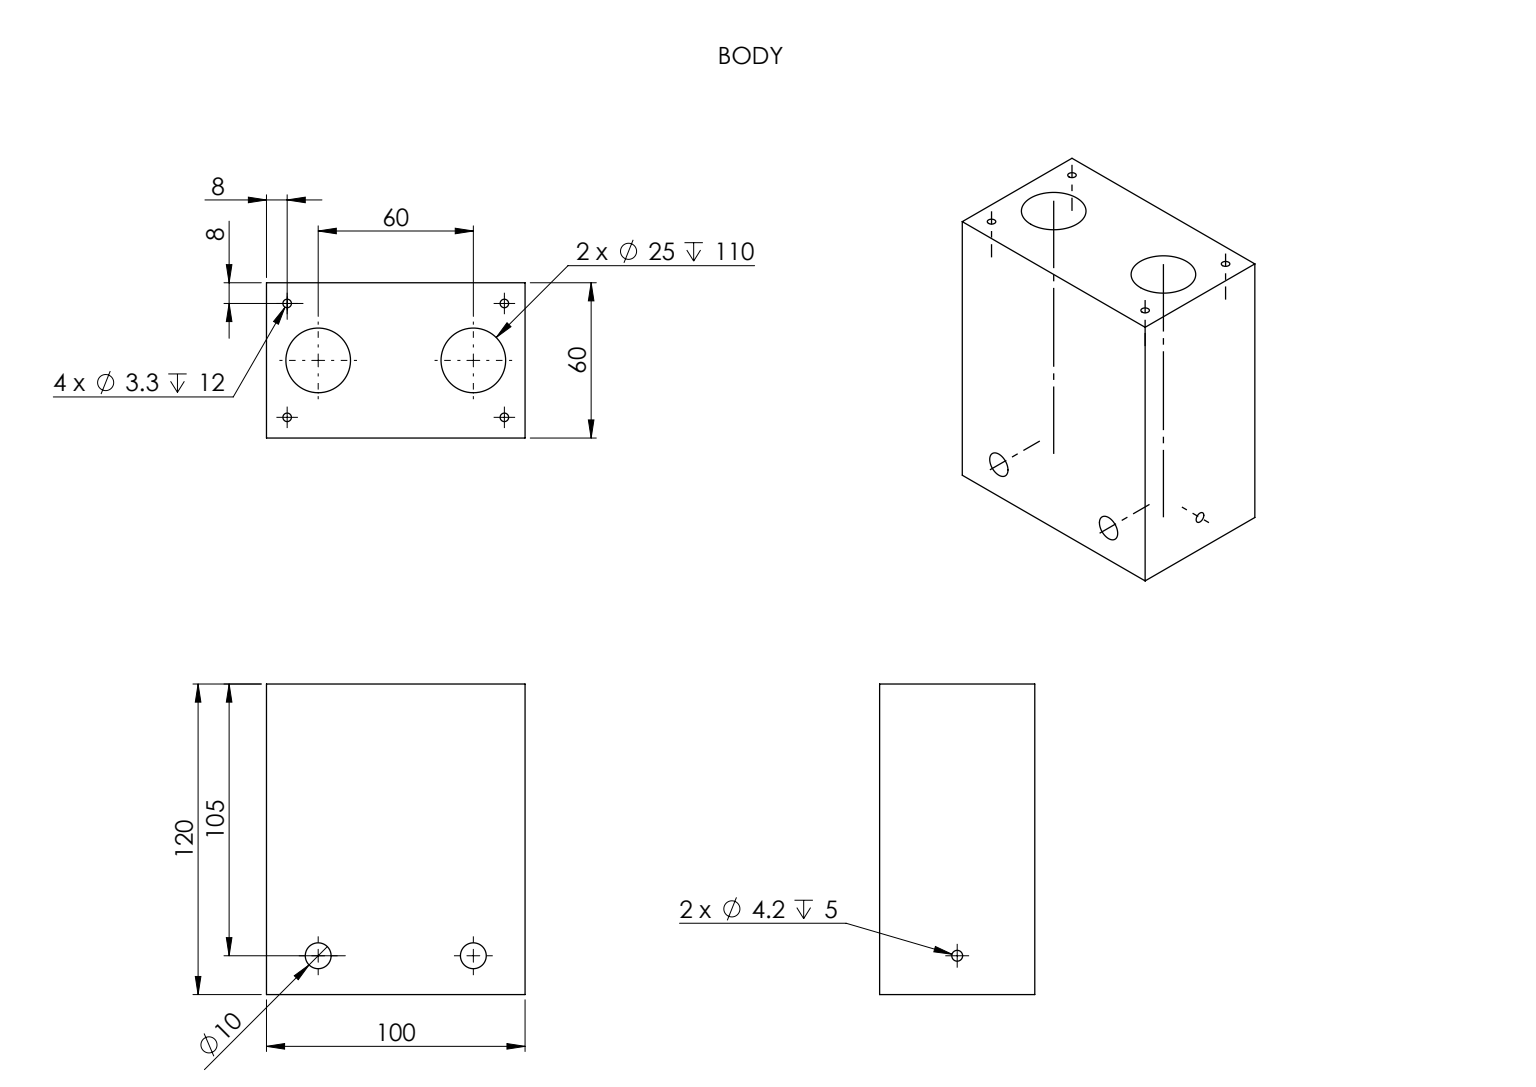
ISO-10303-21;
HEADER;
FILE_DESCRIPTION (('STEP AP214'),
    '1' );
FILE_NAME ('Body.step',
    '2026-09-29T11:11:29',
    ( '' ),
    ( '' ),
    'SwSTEP 2.0',
    'SolidWorks 2026',
    '' );
FILE_SCHEMA (( 'AUTOMOTIVE_DESIGN' ));
ENDSEC;

DATA;
#5=CARTESIAN_POINT ( 'NONE',  ( 42.00000000000000711, 48.00000000000002842, -23.64999999999992042 ) ) ;
#32=CIRCLE ( 'NONE', #4965, 12.49999999999997335 ) ;
#39=STYLED_ITEM ( 'NONE', ( #683 ), #2810 ) ;
#44=CARTESIAN_POINT ( 'NONE',  ( 25.66305258423476943, -47.50955795526802206, 11.72510588894413530 ) ) ;
#45=CARTESIAN_POINT ( 'NONE',  ( -41.99999999999996447, 48.00000000000002842, 22.00000000000000000 ) ) ;
#46=CONICAL_SURFACE ( 'NONE', #7936, 12.49999999999996980, 1.029744258676651869 ) ;
#53=CARTESIAN_POINT ( 'NONE',  ( 26.69566991153659785, -41.23356742411069575, 12.05770814628967535 ) ) ;
#54=DIRECTION ( 'NONE',  ( 1.000000000000000000, 0.000000000000000000, 0.000000000000000000 ) ) ;
#58=VERTEX_POINT ( 'NONE', #8160 ) ;
#70=CARTESIAN_POINT ( 'NONE',  ( -30.00000000000000000, 60.00000000000002842, 0.000000000000000000 ) ) ;
#76=ADVANCED_FACE ( 'NONE', ( #1450 ), #4832, .F. ) ;
#87=ADVANCED_FACE ( 'NONE', ( #4979 ), #2915, .F. ) ;
#90=UNCERTAINTY_MEASURE_WITH_UNIT (LENGTH_MEASURE( 1.000000000000000082E-05 ), #727, 'distance_accuracy_value', 'NONE');
#92=DIRECTION ( 'NONE',  ( -0.000000000000000000, 1.000000000000000000, -0.000000000000000000 ) ) ;
#99=EDGE_CURVE ( 'NONE', #4623, #6070, #4272, .T. ) ;
#100=CARTESIAN_POINT ( 'NONE',  ( -30.00000000000000000, -40.00000000000002132, 12.49999999999998046 ) ) ;
#101=CIRCLE ( 'NONE', #1224, 4.999999999999973355 ) ;
#104=CARTESIAN_POINT ( 'NONE',  ( -49.99999999999997158, -59.99999999999997158, -30.00000000000000000 ) ) ;
#113=ORIENTED_EDGE ( 'NONE', *, *, #1064, .F. ) ;
#125=DIRECTION ( 'NONE',  ( -0.000000000000000000, 1.000000000000000000, -0.000000000000000000 ) ) ;
#139=EDGE_LOOP ( 'NONE', ( #1708, #6887, #7126, #967 ) ) ;
#140=CARTESIAN_POINT ( 'NONE',  ( 0.000000000000000000, 0.000000000000000000, -30.00000000000000000 ) ) ;
#144=CARTESIAN_POINT ( 'NONE',  ( -25.51828610110682405, -42.77717578641267693, 11.66923617342549413 ) ) ;
#145=CARTESIAN_POINT ( 'NONE',  ( 45.00000000000003553, -44.99999999999997158, 0.000000000000000000 ) ) ;
#150=EDGE_LOOP ( 'NONE', ( #1097, #2734, #1435, #2240, #218 ) ) ;
#151=LINE ( 'NONE', #8229, #3888 ) ;
#158=EDGE_CURVE ( 'NONE', #8668, #1053, #2208, .T. ) ;
#161=DIRECTION ( 'NONE',  ( 0.000000000000000000, 0.000000000000000000, 1.000000000000000000 ) ) ;
#187=CARTESIAN_POINT ( 'NONE',  ( 29.34107419296792685, -40.03249052150653142, 12.48689449661282858 ) ) ;
#205=CARTESIAN_POINT ( 'NONE',  ( -25.16271839757670747, -46.30802241892378390, 11.52630626327735364 ) ) ;
#207=VERTEX_POINT ( 'NONE', #7881 ) ;
#210=ORIENTED_EDGE ( 'NONE', *, *, #267, .T. ) ;
#218=ORIENTED_EDGE ( 'NONE', *, *, #2863, .T. ) ;
#228=CARTESIAN_POINT ( 'NONE',  ( 25.51351754887333101, -42.76835092305877595, 11.66791272636411847 ) ) ;
#235=CARTESIAN_POINT ( 'NONE',  ( 50.00000000000002842, -44.99999999999997158, 0.000000000000000000 ) ) ;
#236=ORIENTED_EDGE ( 'NONE', *, *, #746, .T. ) ;
#247=CARTESIAN_POINT ( 'NONE',  ( -49.99999999999997158, 60.00000000000002842, 30.00000000000000000 ) ) ;
#249=ORIENTED_EDGE ( 'NONE', *, *, #158, .T. ) ;
#253=ORIENTED_EDGE ( 'NONE', *, *, #4306, .F. ) ;
#260=ORIENTED_EDGE ( 'NONE', *, *, #8374, .T. ) ;
#267=EDGE_CURVE ( 'NONE', #4999, #1695, #7837, .T. ) ;
#268=DIRECTION ( 'NONE',  ( -0.000000000000000000, 1.000000000000000000, -0.000000000000000000 ) ) ;
#279=ORIENTED_EDGE ( 'NONE', *, *, #4946, .T. ) ;
#290=FACE_OUTER_BOUND ( 'NONE', #2679, .T. ) ;
#302=STYLED_ITEM ( 'NONE', ( #2499 ), #2657 ) ;
#313=CARTESIAN_POINT ( 'NONE',  ( 50.00000000000002842, -44.99999999999997158, 0.000000000000000000 ) ) ;
#327=CARTESIAN_POINT ( 'NONE',  ( 42.00000000000000711, 60.00000000000002842, -20.34999999999992326 ) ) ;
#328=CARTESIAN_POINT ( 'NONE',  ( 25.00000000000004263, -44.99999999999995737, 11.45643923738958314 ) ) ;
#337=ORIENTED_EDGE ( 'NONE', *, *, #267, .F. ) ;
#346=ORIENTED_EDGE ( 'NONE', *, *, #5233, .F. ) ;
#349=CARTESIAN_POINT ( 'NONE',  ( 42.00000000000000711, 60.00000000000002842, -21.99999999999992184 ) ) ;
#356=DIRECTION ( 'NONE',  ( 0.000000000000000000, 0.000000000000000000, 1.000000000000000000 ) ) ;
#358=DIRECTION ( 'NONE',  ( -0.000000000000000000, 1.000000000000000000, -0.000000000000000000 ) ) ;
#366=DIRECTION ( 'NONE',  ( 0.000000000000000000, 0.000000000000000000, 1.000000000000000000 ) ) ;
#372=( LENGTH_UNIT ( ) NAMED_UNIT ( * ) SI_UNIT ( .MILLI., .METRE. ) );
#373=ORIENTED_EDGE ( 'NONE', *, *, #4139, .T. ) ;
#383=CONICAL_SURFACE ( 'NONE', #2372, 1.649999999999998579, 1.029744258676653645 ) ;
#395=EDGE_CURVE ( 'NONE', #6859, #7279, #4993, .T. ) ;
#403=CARTESIAN_POINT ( 'NONE',  ( 33.05708889405230622, -41.03022111473440958, 12.12354317000652770 ) ) ;
#414=ORIENTED_EDGE ( 'NONE', *, *, #7534, .T. ) ;
#417=CARTESIAN_POINT ( 'NONE',  ( -30.33426447602078113, -49.99999999999997868, 12.49999999999998046 ) ) ;
#424=ORIENTED_EDGE ( 'NONE', *, *, #7210, .T. ) ;
#429=CYLINDRICAL_SURFACE ( 'NONE', #2354, 1.649999999999998579 ) ;
#433=DIRECTION ( 'NONE',  ( -0.000000000000000000, 1.000000000000000000, -0.000000000000000000 ) ) ;
#443=CARTESIAN_POINT ( 'NONE',  ( 33.76876201869192329, -41.69806059905381090, 11.92074493419279158 ) ) ;
#447=CARTESIAN_POINT ( 'NONE',  ( -50.00000000000002842, -44.99999999999997158, 0.000000000000000000 ) ) ;
#448=COLOUR_RGB ( '', 0.66274510, 0.83137255, 0.94901961) ;
#451=LINE ( 'NONE', #2589, #1885 ) ;
#454=AXIS2_PLACEMENT_3D ( 'NONE', #6879, #842, #8222 ) ;
#458=CARTESIAN_POINT ( 'NONE',  ( -30.66228279038040228, -49.96682304584954437, 12.48662461771948529 ) ) ;
#461=DIRECTION ( 'NONE',  ( -0.000000000000000000, 1.000000000000000000, -0.000000000000000000 ) ) ;
#467=ORIENTED_EDGE ( 'NONE', *, *, #5580, .T. ) ;
#481=VECTOR ( 'NONE', #6597, 1000.000000000000000 ) ;
#491=ORIENTED_EDGE ( 'NONE', *, *, #6060, .T. ) ;
#495=EDGE_CURVE ( 'NONE', #3168, #8538, #1819, .T. ) ;
#498=ORIENTED_EDGE ( 'NONE', *, *, #6490, .F. ) ;
#500=CARTESIAN_POINT ( 'NONE',  ( -34.82961390090871134, -46.30459253935130448, 11.52942094433410425 ) ) ;
#518=CARTESIAN_POINT ( 'NONE',  ( -41.99999999999996447, 48.00000000000002842, 20.35000000000000142 ) ) ;
#523=ORIENTED_EDGE ( 'NONE', *, *, #1974, .F. ) ;
#529=CARTESIAN_POINT ( 'NONE',  ( 30.00000000000000000, -49.99999999999997158, -1.102182119232617753E-14 ) ) ;
#533=ADVANCED_FACE ( 'NONE', ( #4459 ), #1022, .F. ) ;
#534=CARTESIAN_POINT ( 'NONE',  ( 30.00000000000000000, 60.00000000000002842, -1.102182119232617753E-14 ) ) ;
#548=CARTESIAN_POINT ( 'NONE',  ( 33.76617411639087152, -48.30471456237972205, 11.92153802757354342 ) ) ;
#550=EDGE_LOOP ( 'NONE', ( #7307, #8387, #6188 ) ) ;
#556=B_SPLINE_CURVE_WITH_KNOTS ( 'NONE', 3,
 ( #4547, #3887, #5995, #8125, #5416, #2084, #2749, #4769, #1411, #7454, #4108, #44, #6786, #749, #6087, #3810, #3729, #1657, #2452, #328 ),
 .UNSPECIFIED., .F., .F.,
 ( 4, 2, 2, 2, 2, 2, 2, 2, 2, 4 ),
 ( 2.088883680402604765E-17, 0.0009878455431464048045, 0.001975691086292788792, 0.002963536629439172780, 0.003951382172585556768, 0.004939227715731940756, 0.005927073258878324744, 0.006420996030451506763, 0.006914918802024689649, 0.007902764345171071902 ),
 .UNSPECIFIED. ) ;
#567=EDGE_LOOP ( 'NONE', ( #498, #2058, #5139, #6935, #113, #2462 ) ) ;
#579=AXIS2_PLACEMENT_3D ( 'NONE', #3617, #8335, #2961 ) ;
#589=MECHANICAL_DESIGN_GEOMETRIC_PRESENTATION_REPRESENTATION('',(#39),#3149);
#597=VECTOR ( 'NONE', #1210, 1000.000000000000000 ) ;
#605=VECTOR ( 'NONE', #8413, 1000.000000000000000 ) ;
#620=DIRECTION ( 'NONE',  ( -0.000000000000000000, 1.000000000000000000, -0.000000000000000000 ) ) ;
#625=EDGE_LOOP ( 'NONE', ( #5700, #4753, #2629, #4443 ) ) ;
#626=CARTESIAN_POINT ( 'NONE',  ( -50.00000000000002842, -44.99999999999997158, 2.099999999999997868 ) ) ;
#637=FILL_AREA_STYLE_COLOUR ( '', #448 ) ;
#638=LINE ( 'NONE', #4044, #1797 ) ;
#645=CIRCLE ( 'NONE', #5579, 1.649999999999998579 ) ;
#654=AXIS2_PLACEMENT_3D ( 'NONE', #7280, #754, #5374 ) ;
#668=DIRECTION ( 'NONE',  ( 0.000000000000000000, 0.000000000000000000, -1.000000000000000000 ) ) ;
#671=DIRECTION ( 'NONE',  ( -0.000000000000000000, 1.000000000000000000, -0.000000000000000000 ) ) ;
#674=LINE ( 'NONE', #8046, #3482 ) ;
#679=CLOSED_SHELL ( 'NONE', ( #7354, #6229, #8350, #1433, #4093, #6520, #7720, #1560, #7628, #4521, #4016, #3800, #5743, #3822, #7621, #4055, #7669, #4185, #6558, #1536, #3196, #3679, #1549, #5972, #76, #87, #7313, #7419, #7801, #4973, #8008, #2481, #4022, #3615, #4856, #2349, #5957, #8496, #3760, #533, #2845, #7262 ) ) ;
#683=PRESENTATION_STYLE_ASSIGNMENT (( #2596 ) ) ;
#686=CARTESIAN_POINT ( 'NONE',  ( 32.51701891408353617, -49.33233869400790184, 12.24706002614420264 ) ) ;
#699=CONICAL_SURFACE ( 'NONE', #7040, 12.49999999999997335, 1.029744258676651869 ) ;
#708=DIRECTION ( 'NONE',  ( 1.049727191138618079E-16, 0.5150380749100549327, -0.8571673007021118895 ) ) ;
#711=CARTESIAN_POINT ( 'NONE',  ( -41.99999999999996447, 47.00857997860455129, -22.00000000000000000 ) ) ;
#712=DIRECTION ( 'NONE',  ( 0.000000000000000000, 0.000000000000000000, 1.000000000000000000 ) ) ;
#724=VERTEX_POINT ( 'NONE', #2388 ) ;
#727=( LENGTH_UNIT ( ) NAMED_UNIT ( * ) SI_UNIT ( .MILLI., .METRE. ) );
#728=DIRECTION ( 'NONE',  ( 1.049727191138617093E-16, 0.5150380749100563760, -0.8571673007021110013 ) ) ;
#735=EDGE_CURVE ( 'NONE', #1784, #5916, #4447, .T. ) ;
#739=DIRECTION ( 'NONE',  ( 0.000000000000000000, 0.000000000000000000, 1.000000000000000000 ) ) ;
#746=EDGE_CURVE ( 'NONE', #2486, #6385, #6425, .T. ) ;
#749=CARTESIAN_POINT ( 'NONE',  ( 25.32221232802729460, -46.77334385938312522, 11.59192968702632065 ) ) ;
#754=DIRECTION ( 'NONE',  ( -0.000000000000000000, -0.000000000000000000, 1.000000000000000000 ) ) ;
#759=FACE_OUTER_BOUND ( 'NONE', #5969, .T. ) ;
#762=CYLINDRICAL_SURFACE ( 'NONE', #8087, 1.649999999999998579 ) ;
#766=EDGE_LOOP ( 'NONE', ( #3607, #2663 ) ) ;
#778=EDGE_CURVE ( 'NONE', #6845, #1128, #7172, .T. ) ;
#784=DIRECTION ( 'NONE',  ( 0.000000000000000000, 0.000000000000000000, 1.000000000000000000 ) ) ;
#801=VECTOR ( 'NONE', #7421, 1000.000000000000000 ) ;
#803=EDGE_CURVE ( 'NONE', #4035, #3309, #1727, .T. ) ;
#805=CARTESIAN_POINT ( 'NONE',  ( 29.67102067851989844, -40.00000000000000000, 12.49999999999996980 ) ) ;
#820=LINE ( 'NONE', #2774, #3625 ) ;
#823=FACE_BOUND ( 'NONE', #7168, .T. ) ;
#829=DIRECTION ( 'NONE',  ( 0.000000000000000000, 0.000000000000000000, 1.000000000000000000 ) ) ;
#842=DIRECTION ( 'NONE',  ( 0.000000000000000000, 0.000000000000000000, 1.000000000000000000 ) ) ;
#845=CARTESIAN_POINT ( 'NONE',  ( 25.16326641152763344, -43.69081521296084958, 11.52653374317613455 ) ) ;
#846=DIRECTION ( 'NONE',  ( -0.000000000000000000, 1.000000000000000000, -0.000000000000000000 ) ) ;
#857=AXIS2_PLACEMENT_3D ( 'NONE', #3752, #2969, #5644 ) ;
#868=EDGE_LOOP ( 'NONE', ( #8063, #1620, #467 ) ) ;
#880=VECTOR ( 'NONE', #8032, 1000.000000000000000 ) ;
#883=CARTESIAN_POINT ( 'NONE',  ( -30.00000000000000000, 60.00000000000002842, 12.49999999999998757 ) ) ;
#884=PRODUCT_CONTEXT ( 'NONE', #2293, 'mechanical' ) ;
#885=CARTESIAN_POINT ( 'NONE',  ( -41.99999999999996447, 48.00000000000002842, -23.64999999999999858 ) ) ;
#897=EDGE_LOOP ( 'NONE', ( #6623, #5315 ) ) ;
#906=DIRECTION ( 'NONE',  ( -1.000000000000000000, -0.000000000000000000, -0.000000000000000000 ) ) ;
#907=CARTESIAN_POINT ( 'NONE',  ( -34.33209868862994796, -42.48249851487850748, 11.72687238757476003 ) ) ;
#911=EDGE_CURVE ( 'NONE', #6845, #2769, #1890, .T. ) ;
#912=VERTEX_POINT ( 'NONE', #6680 ) ;
#915=ORIENTED_EDGE ( 'NONE', *, *, #5570, .F. ) ;
#919=LINE ( 'NONE', #1532, #6968 ) ;
#925=CIRCLE ( 'NONE', #7677, 1.649999999999998579 ) ;
#935=CARTESIAN_POINT ( 'NONE',  ( -26.02663761693602495, -41.94765302695305564, 11.85321826485150432 ) ) ;
#947=CIRCLE ( 'NONE', #3762, 1.649999999999998579 ) ;
#962=DIRECTION ( 'NONE',  ( -1.000000000000000000, -0.000000000000000000, -0.000000000000000000 ) ) ;
#967=ORIENTED_EDGE ( 'NONE', *, *, #158, .F. ) ;
#971=CARTESIAN_POINT ( 'NONE',  ( -41.99999999999996447, 60.00000000000002842, 20.35000000000000142 ) ) ;
#983=ORIENTED_EDGE ( 'NONE', *, *, #2920, .F. ) ;
#988=B_SPLINE_CURVE_WITH_KNOTS ( 'NONE', 3,
 ( #3772, #7077, #5751, #3162, #1036, #2329, #5007, #7696, #3075, #403, #8450, #443, #5836, #2492, #5173, #4512, #8089, #7329, #1955, #5292, #8613, #1873 ),
 .UNSPECIFIED., .F., .F.,
 ( 4, 2, 2, 2, 2, 2, 2, 2, 2, 2, 4 ),
 ( 0.01579945264986103853, 0.01629290087626464323, 0.01678634910266824792, 0.01777324555547545731, 0.01876014200828266323, 0.01974703846108986915, 0.02073393491389707508, 0.02122738314030068324, 0.02172083136670428793, 0.02270772781951150079, 0.02369462427231871365 ),
 .UNSPECIFIED. ) ;
#991=DIRECTION ( 'NONE',  ( -0.000000000000000000, 1.000000000000000000, -0.000000000000000000 ) ) ;
#992=CARTESIAN_POINT ( 'NONE',  ( -26.23382588360912848, -48.30471456237976469, 11.92153802757356118 ) ) ;
#995=EDGE_CURVE ( 'NONE', #5982, #8204, #1392, .T. ) ;
#1005=DIRECTION ( 'NONE',  ( -1.000000000000000000, 0.000000000000000000, 0.000000000000000000 ) ) ;
#1008=EDGE_CURVE ( 'NONE', #6235, #8538, #3206, .T. ) ;
#1016=CIRCLE ( 'NONE', #1730, 12.49999999999998401 ) ;
#1018=EDGE_CURVE ( 'NONE', #2059, #1305, #638, .T. ) ;
#1022=CYLINDRICAL_SURFACE ( 'NONE', #3219, 2.099999999999997868 ) ;
#1024=DIRECTION ( 'NONE',  ( 0.000000000000000000, 0.000000000000000000, 1.000000000000000000 ) ) ;
#1026=LINE ( 'NONE', #3103, #1095 ) ;
#1029=ORIENTED_EDGE ( 'NONE', *, *, #2094, .F. ) ;
#1036=CARTESIAN_POINT ( 'NONE',  ( 30.82435085130693153, -40.06565635038678863, 12.47384660903967735 ) ) ;
#1049=CYLINDRICAL_SURFACE ( 'NONE', #6547, 1.649999999999998579 ) ;
#1051=CARTESIAN_POINT ( 'NONE',  ( 50.00000000000002842, -59.99999999999997158, 30.00000000000000000 ) ) ;
#1053=VERTEX_POINT ( 'NONE', #2859 ) ;
#1055=EDGE_CURVE ( 'NONE', #6557, #4874, #820, .T. ) ;
#1062=PRODUCT ( 'Body', 'Body', '', ( #884 ) ) ;
#1064=EDGE_CURVE ( 'NONE', #7279, #8149, #6180, .T. ) ;
#1067=CARTESIAN_POINT ( 'NONE',  ( 42.00000000000000711, 48.00000000000002842, 21.99999999999992184 ) ) ;
#1069=DIRECTION ( 'NONE',  ( 0.000000000000000000, 0.000000000000000000, 1.000000000000000000 ) ) ;
#1076=VECTOR ( 'NONE', #3796, 1000.000000000000000 ) ;
#1081=CARTESIAN_POINT ( 'NONE',  ( -49.99999999999997158, -59.99999999999997158, 30.00000000000000000 ) ) ;
#1089=VECTOR ( 'NONE', #1578, 1000.000000000000000 ) ;
#1091=CARTESIAN_POINT ( 'NONE',  ( -30.00000000000000000, -49.99999999999997158, 12.49999999999997335 ) ) ;
#1095=VECTOR ( 'NONE', #5784, 1000.000000000000000 ) ;
#1097=ORIENTED_EDGE ( 'NONE', *, *, #3505, .F. ) ;
#1100=VERTEX_POINT ( 'NONE', #4132 ) ;
#1121=CARTESIAN_POINT ( 'NONE',  ( -26.02892847301724544, -48.05549307397419767, 11.85400291056945576 ) ) ;
#1124=EDGE_LOOP ( 'NONE', ( #7069, #6657, #3793 ) ) ;
#1128=VERTEX_POINT ( 'NONE', #4173 ) ;
#1134=CARTESIAN_POINT ( 'NONE',  ( 42.00000000000000711, 48.00000000000002842, -20.34999999999992326 ) ) ;
#1142=DIRECTION ( 'NONE',  ( 0.000000000000000000, 0.000000000000000000, 1.000000000000000000 ) ) ;
#1152=EDGE_LOOP ( 'NONE', ( #2553, #2380, #260, #2838 ) ) ;
#1165=CIRCLE ( 'NONE', #5378, 4.999999999999969802 ) ;
#1173=ORIENTED_EDGE ( 'NONE', *, *, #7210, .F. ) ;
#1176=CARTESIAN_POINT ( 'NONE',  ( -34.99999999999997868, -45.33027059730886066, 11.45643923738958847 ) ) ;
#1179=DIRECTION ( 'NONE',  ( 1.049727191138617093E-16, 0.5150380749100563760, -0.8571673007021110013 ) ) ;
#1187=CARTESIAN_POINT ( 'NONE',  ( 30.00000000000001421, -49.99999999999997158, 12.49999999999995914 ) ) ;
#1190=CARTESIAN_POINT ( 'NONE',  ( -34.99999999999997868, -45.00000000000000000, 11.45643923738958847 ) ) ;
#1201=DIRECTION ( 'NONE',  ( -0.5150380749100560429, 1.049727191138617340E-16, -0.8571673007021112234 ) ) ;
#1206=CARTESIAN_POINT ( 'NONE',  ( 30.00000000000000000, 60.00000000000002842, -1.102182119232617753E-14 ) ) ;
#1210=DIRECTION ( 'NONE',  ( 0.000000000000000000, 0.5150380749100549327, 0.8571673007021118895 ) ) ;
#1224=AXIS2_PLACEMENT_3D ( 'NONE', #5201, #3231, #6698 ) ;
#1225=EDGE_LOOP ( 'NONE', ( #7122, #8635, #4534, #6637, #1029, #5348 ) ) ;
#1236=CARTESIAN_POINT ( 'NONE',  ( -49.99999999999997158, -59.99999999999997158, -30.00000000000000000 ) ) ;
#1238=ORIENTED_EDGE ( 'NONE', *, *, #4139, .F. ) ;
#1242=CARTESIAN_POINT ( 'NONE',  ( -50.00000000000002842, -44.99999999999997158, 0.000000000000000000 ) ) ;
#1246=CARTESIAN_POINT ( 'NONE',  ( 42.00000000000000711, 60.00000000000002842, 21.99999999999992184 ) ) ;
#1253=ORIENTED_EDGE ( 'NONE', *, *, #4029, .F. ) ;
#1257=DIRECTION ( 'NONE',  ( -0.000000000000000000, 1.000000000000000000, -0.000000000000000000 ) ) ;
#1260=ORIENTED_EDGE ( 'NONE', *, *, #4573, .F. ) ;
#1278=ORIENTED_EDGE ( 'NONE', *, *, #3659, .T. ) ;
#1290=ORIENTED_EDGE ( 'NONE', *, *, #3181, .F. ) ;
#1303=CARTESIAN_POINT ( 'NONE',  ( 33.97107152698276877, -48.05549307397414793, 11.85400291056944333 ) ) ;
#1305=VERTEX_POINT ( 'NONE', #5506 ) ;
#1317=AXIS2_PLACEMENT_3D ( 'NONE', #1754, #3775, #7828 ) ;
#1324=CARTESIAN_POINT ( 'NONE',  ( 30.00000000000000000, 60.00000000000002842, -12.49999999999999467 ) ) ;
#1344=SURFACE_SIDE_STYLE ('',( #6065 ) ) ;
#1347=CARTESIAN_POINT ( 'NONE',  ( -30.00000000000000000, -49.99999999999997158, 12.49999999999997335 ) ) ;
#1354=VERTEX_POINT ( 'NONE', #971 ) ;
#1365=B_SPLINE_CURVE_WITH_KNOTS ( 'NONE', 3,
 ( #100, #6269, #6969, #8177, #4869, #4159, #5558, #4243, #4776, #6926, #3506, #5604, #935, #6183, #2889, #144, #5516, #5425, #8225, #8134, #2093, #4377 ),
 .UNSPECIFIED., .F., .F.,
 ( 4, 2, 2, 2, 2, 2, 2, 2, 2, 2, 4 ),
 ( 0.01579945264986107323, 0.01629290087626467792, 0.01678634910266828609, 0.01777324555547549201, 0.01876014200828270140, 0.01974703846108990732, 0.02073393491389711671, 0.02122738314030071100, 0.02172083136670430875, 0.02270772781951152161, 0.02369462427231873447 ),
 .UNSPECIFIED. ) ;
#1372=CYLINDRICAL_SURFACE ( 'NONE', #654, 4.999999999999973355 ) ;
#1379=CARTESIAN_POINT ( 'NONE',  ( 42.00000000000000711, 48.00000000000002842, 21.99999999999992184 ) ) ;
#1382=ORIENTED_EDGE ( 'NONE', *, *, #5368, .F. ) ;
#1392=LINE ( 'NONE', #8630, #8276 ) ;
#1400=ORIENTED_EDGE ( 'NONE', *, *, #3769, .F. ) ;
#1401=EDGE_LOOP ( 'NONE', ( #1260, #6461 ) ) ;
#1411=CARTESIAN_POINT ( 'NONE',  ( 26.68912794345745709, -48.76061935842967898, 12.05589577412331082 ) ) ;
#1412=CARTESIAN_POINT ( 'NONE',  ( 42.00000000000000711, 60.00000000000002842, 20.34999999999992326 ) ) ;
#1420=CARTESIAN_POINT ( 'NONE',  ( 25.00000000000004619, -44.66998333124461595, 11.45643923738958314 ) ) ;
#1422=FACE_OUTER_BOUND ( 'NONE', #4365, .T. ) ;
#1433=ADVANCED_FACE ( 'NONE', ( #2687 ), #7405, .F. ) ;
#1435=ORIENTED_EDGE ( 'NONE', *, *, #5478, .T. ) ;
#1450=FACE_OUTER_BOUND ( 'NONE', #5373, .T. ) ;
#1465=CARTESIAN_POINT ( 'NONE',  ( 27.49109988343930766, -40.67193172067894835, 12.24650812517141674 ) ) ;
#1479=CARTESIAN_POINT ( 'NONE',  ( -32.22066341043710480, -40.51720970344483419, 12.30204028087673862 ) ) ;
#1483=EDGE_LOOP ( 'NONE', ( #1839, #1601, #3000 ) ) ;
#1499=CARTESIAN_POINT ( 'NONE',  ( -41.99999999999996447, 60.00000000000002842, 20.35000000000000142 ) ) ;
#1501=ORIENTED_EDGE ( 'NONE', *, *, #5685, .F. ) ;
#1507=CARTESIAN_POINT ( 'NONE',  ( 26.02887806073490751, -41.94466314146772845, 11.85397847079113731 ) ) ;
#1509=FACE_OUTER_BOUND ( 'NONE', #7442, .T. ) ;
#1525=PLANE ( 'NONE',  #3187 ) ;
#1526=ORIENTED_EDGE ( 'NONE', *, *, #6608, .F. ) ;
#1529=ORIENTED_EDGE ( 'NONE', *, *, #3755, .F. ) ;
#1531=CARTESIAN_POINT ( 'NONE',  ( 42.00000000000000711, 60.00000000000002842, 23.64999999999992042 ) ) ;
#1532=CARTESIAN_POINT ( 'NONE',  ( -50.00000000000002842, -44.99999999999997158, -2.099999999999997868 ) ) ;
#1536=ADVANCED_FACE ( 'NONE', ( #4843, #4796, #4135, #4219, #5577, #4091, #6201 ), #4925, .F. ) ;
#1539=EDGE_CURVE ( 'NONE', #8159, #6416, #3611, .T. ) ;
#1546=EDGE_CURVE ( 'NONE', #4874, #8668, #2062, .T. ) ;
#1548=CIRCLE ( 'NONE', #2830, 1.649999999999998579 ) ;
#1549=ADVANCED_FACE ( 'NONE', ( #823, #2909, #4176 ), #1525, .F. ) ;
#1555=DIRECTION ( 'NONE',  ( 0.000000000000000000, 0.000000000000000000, 1.000000000000000000 ) ) ;
#1560=ADVANCED_FACE ( 'NONE', ( #1568 ), #2357, .F. ) ;
#1565=CARTESIAN_POINT ( 'NONE',  ( -32.07348704419703012, -40.44729329317338795, 12.32776405682971621 ) ) ;
#1568=FACE_OUTER_BOUND ( 'NONE', #1483, .T. ) ;
#1578=DIRECTION ( 'NONE',  ( 1.000000000000000000, 0.000000000000000000, 0.000000000000000000 ) ) ;
#1598=VECTOR ( 'NONE', #3859, 1000.000000000000000 ) ;
#1601=ORIENTED_EDGE ( 'NONE', *, *, #5761, .T. ) ;
#1602=CARTESIAN_POINT ( 'NONE',  ( 50.00000000000002842, -59.99999999999997158, 30.00000000000000000 ) ) ;
#1614=CARTESIAN_POINT ( 'NONE',  ( -26.94596629111760322, -48.97208017019580950, 12.12430375744701827 ) ) ;
#1617=VERTEX_POINT ( 'NONE', #5442 ) ;
#1620=ORIENTED_EDGE ( 'NONE', *, *, #6650, .T. ) ;
#1622=DIRECTION ( 'NONE',  ( -0.000000000000000000, 1.000000000000000000, -0.000000000000000000 ) ) ;
#1623=FACE_OUTER_BOUND ( 'NONE', #5831, .T. ) ;
#1625=CARTESIAN_POINT ( 'NONE',  ( -30.00000000000000000, 60.00000000000002842, -12.49999999999998934 ) ) ;
#1636=CARTESIAN_POINT ( 'NONE',  ( 30.00000000000000000, -49.99999999999997158, -12.49999999999998046 ) ) ;
#1638=AXIS2_PLACEMENT_3D ( 'NONE', #235, #8314, #8308 ) ;
#1643=DIRECTION ( 'NONE',  ( -0.000000000000000000, 1.000000000000000000, -0.000000000000000000 ) ) ;
#1645=DIRECTION ( 'NONE',  ( 1.000000000000000000, 0.000000000000000000, 0.000000000000000000 ) ) ;
#1648=ORIENTED_EDGE ( 'NONE', *, *, #803, .T. ) ;
#1657=CARTESIAN_POINT ( 'NONE',  ( 25.03240331249625328, -45.65721116879221597, 11.47074269425085191 ) ) ;
#1667=ORIENTED_EDGE ( 'NONE', *, *, #1064, .T. ) ;
#1669=CARTESIAN_POINT ( 'NONE',  ( -32.51667136668694269, -49.33273298888241243, 12.24717930254582043 ) ) ;
#1672=CARTESIAN_POINT ( 'NONE',  ( 42.00000000000000711, 60.00000000000002842, -21.99999999999992184 ) ) ;
#1673=CARTESIAN_POINT ( 'NONE',  ( 30.00000000000000000, 60.00000000000002842, -12.49999999999998757 ) ) ;
#1677=EDGE_LOOP ( 'NONE', ( #5190, #1290, #7369, #3341, #3312, #2576 ) ) ;
#1680=DIRECTION ( 'NONE',  ( -1.000000000000000000, -0.000000000000000000, -0.000000000000000000 ) ) ;
#1688=CARTESIAN_POINT ( 'NONE',  ( 42.00000000000000711, 60.00000000000002842, -20.34999999999992326 ) ) ;
#1692=EDGE_CURVE ( 'NONE', #6529, #4035, #5048, .T. ) ;
#1695=VERTEX_POINT ( 'NONE', #5090 ) ;
#1699=VECTOR ( 'NONE', #4425, 1000.000000000000000 ) ;
#1700=DIRECTION ( 'NONE',  ( -0.000000000000000000, 1.000000000000000000, -0.000000000000000000 ) ) ;
#1705=CARTESIAN_POINT ( 'NONE',  ( -30.00000000000000000, -49.99999999999997158, 12.49999999999997335 ) ) ;
#1707=DIRECTION ( 'NONE',  ( 0.000000000000000000, 0.000000000000000000, 1.000000000000000000 ) ) ;
#1708=ORIENTED_EDGE ( 'NONE', *, *, #1546, .F. ) ;
#1713=VERTEX_POINT ( 'NONE', #8449 ) ;
#1716=DIRECTION ( 'NONE',  ( -0.000000000000000000, 1.000000000000000000, -0.000000000000000000 ) ) ;
#1724=PRODUCT_DEFINITION_FORMATION_WITH_SPECIFIED_SOURCE ( 'ANY', '', #1062, .NOT_KNOWN. ) ;
#1725=ORIENTED_EDGE ( 'NONE', *, *, #7252, .T. ) ;
#1727=CIRCLE ( 'NONE', #8211, 1.649999999999998579 ) ;
#1730=AXIS2_PLACEMENT_3D ( 'NONE', #3712, #5159, #5825 ) ;
#1738=FACE_OUTER_BOUND ( 'NONE', #5933, .T. ) ;
#1740=CARTESIAN_POINT ( 'NONE',  ( -49.99999999999997158, 60.00000000000002842, 30.00000000000000000 ) ) ;
#1754=CARTESIAN_POINT ( 'NONE',  ( -50.00000000000002842, -44.99999999999997158, 0.000000000000000000 ) ) ;
#1784=VERTEX_POINT ( 'NONE', #711 ) ;
#1796=CARTESIAN_POINT ( 'NONE',  ( -25.00000000000002487, -45.00000000000000000, 30.00000000000000000 ) ) ;
#1797=VECTOR ( 'NONE', #6632, 1000.000000000000000 ) ;
#1806=CARTESIAN_POINT ( 'NONE',  ( -41.99999999999996447, 48.00000000000002842, -23.64999999999999858 ) ) ;
#1809=ORIENTED_EDGE ( 'NONE', *, *, #3323, .T. ) ;
#1815=FACE_OUTER_BOUND ( 'NONE', #4053, .T. ) ;
#1816=DIRECTION ( 'NONE',  ( -0.5150380749100560429, 0.000000000000000000, 0.8571673007021112234 ) ) ;
#1819=LINE ( 'NONE', #518, #4339 ) ;
#1820=DIRECTION ( 'NONE',  ( 0.000000000000000000, 0.000000000000000000, 1.000000000000000000 ) ) ;
#1834=CYLINDRICAL_SURFACE ( 'NONE', #3445, 12.49999999999997691 ) ;
#1839=ORIENTED_EDGE ( 'NONE', *, *, #2379, .F. ) ;
#1873=CARTESIAN_POINT ( 'NONE',  ( 34.99999999999998579, -44.99999999999995737, 11.45643923738957071 ) ) ;
#1876=DIRECTION ( 'NONE',  ( -0.000000000000000000, 1.000000000000000000, -0.000000000000000000 ) ) ;
#1881=LINE ( 'NONE', #4566, #597 ) ;
#1884=EDGE_CURVE ( 'NONE', #724, #2594, #7698, .T. ) ;
#1885=VECTOR ( 'NONE', #2541, 1000.000000000000000 ) ;
#1889=CARTESIAN_POINT ( 'NONE',  ( 30.00000000000000000, -39.99999999999998579, 12.49999999999996625 ) ) ;
#1890=LINE ( 'NONE', #7345, #2857 ) ;
#1916=DIRECTION ( 'NONE',  ( 0.000000000000000000, 0.000000000000000000, 1.000000000000000000 ) ) ;
#1920=ORIENTED_EDGE ( 'NONE', *, *, #1055, .F. ) ;
#1924=EDGE_CURVE ( 'NONE', #6529, #7164, #925, .T. ) ;
#1927=ORIENTED_EDGE ( 'NONE', *, *, #7948, .F. ) ;
#1937=EDGE_CURVE ( 'NONE', #6055, #4623, #6616, .T. ) ;
#1951=FACE_OUTER_BOUND ( 'NONE', #4537, .T. ) ;
#1955=CARTESIAN_POINT ( 'NONE',  ( 34.83675056951057059, -43.69086006543227541, 11.52652666073311316 ) ) ;
#1958=DIRECTION ( 'NONE',  ( -0.000000000000000000, 1.000000000000000000, -0.000000000000000000 ) ) ;
#1974=EDGE_CURVE ( 'NONE', #5482, #1354, #5414, .T. ) ;
#1995=LINE ( 'NONE', #6136, #7420 ) ;
#1999=DIRECTION ( 'NONE',  ( -0.000000000000000000, -0.000000000000000000, -1.000000000000000000 ) ) ;
#2006=CIRCLE ( 'NONE', #579, 1.649999999999998579 ) ;
#2013=VECTOR ( 'NONE', #92, 1000.000000000000000 ) ;
#2022=EDGE_LOOP ( 'NONE', ( #6847, #3430 ) ) ;
#2040=ORIENTED_EDGE ( 'NONE', *, *, #2379, .T. ) ;
#2045=CARTESIAN_POINT ( 'NONE',  ( 42.00000000000000711, 48.00000000000002842, -21.99999999999992184 ) ) ;
#2046=CARTESIAN_POINT ( 'NONE',  ( -25.00000000000002487, -45.00000000000000000, -30.00100000000000122 ) ) ;
#2058=ORIENTED_EDGE ( 'NONE', *, *, #2254, .T. ) ;
#2059=VERTEX_POINT ( 'NONE', #2931 ) ;
#2061=FACE_OUTER_BOUND ( 'NONE', #7222, .T. ) ;
#2062=CIRCLE ( 'NONE', #6979, 1.649999999999998579 ) ;
#2067=ORIENTED_EDGE ( 'NONE', *, *, #746, .F. ) ;
#2068=CIRCLE ( 'NONE', #6142, 2.099999999999997868 ) ;
#2084=CARTESIAN_POINT ( 'NONE',  ( 27.76939715822961219, -49.48683715626706459, 12.30316928347422412 ) ) ;
#2089=DIRECTION ( 'NONE',  ( -0.000000000000000000, 1.000000000000000000, -0.000000000000000000 ) ) ;
#2093=CARTESIAN_POINT ( 'NONE',  ( -25.00000000000001776, -44.67046583110986546, 11.45643923738959025 ) ) ;
#2094=EDGE_CURVE ( 'NONE', #4829, #2602, #7056, .T. ) ;
#2095=DIRECTION ( 'NONE',  ( 0.000000000000000000, 0.000000000000000000, -1.000000000000000000 ) ) ;
#2103=EDGE_CURVE ( 'NONE', #8149, #1617, #1365, .T. ) ;
#2114=DIRECTION ( 'NONE',  ( 0.000000000000000000, -0.000000000000000000, -1.000000000000000000 ) ) ;
#2119=VECTOR ( 'NONE', #5796, 1000.000000000000000 ) ;
#2135=ORIENTED_EDGE ( 'NONE', *, *, #4306, .T. ) ;
#2136=FACE_OUTER_BOUND ( 'NONE', #2557, .T. ) ;
#2139=DIRECTION ( 'NONE',  ( -0.000000000000000000, 1.000000000000000000, -0.000000000000000000 ) ) ;
#2143=DIRECTION ( 'NONE',  ( 0.000000000000000000, 0.000000000000000000, 1.000000000000000000 ) ) ;
#2152=VECTOR ( 'NONE', #1179, 1000.000000000000000 ) ;
#2153=LINE ( 'NONE', #4839, #8074 ) ;
#2174=DIRECTION ( 'NONE',  ( 0.000000000000000000, 0.5150380749100563760, 0.8571673007021110013 ) ) ;
#2199=CARTESIAN_POINT ( 'NONE',  ( -25.00000000000002487, -45.00000000000000000, 11.45643923738959025 ) ) ;
#2200=VECTOR ( 'NONE', #1999, 1000.000000000000000 ) ;
#2206=ORIENTED_EDGE ( 'NONE', *, *, #2771, .T. ) ;
#2208=LINE ( 'NONE', #1531, #8280 ) ;
#2212=CARTESIAN_POINT ( 'NONE',  ( -30.00000000000000000, -49.99999999999997158, -12.49999999999997335 ) ) ;
#2227=CARTESIAN_POINT ( 'NONE',  ( 25.25924940455542611, -43.37701935357445393, 11.56693546130993155 ) ) ;
#2235=ORIENTED_EDGE ( 'NONE', *, *, #3215, .T. ) ;
#2240=ORIENTED_EDGE ( 'NONE', *, *, #7070, .T. ) ;
#2253=CARTESIAN_POINT ( 'NONE',  ( 42.00000000000000711, 48.00000000000002842, -20.34999999999992326 ) ) ;
#2254=EDGE_CURVE ( 'NONE', #6385, #6416, #5740, .T. ) ;
#2263=VECTOR ( 'NONE', #5559, 1000.000000000000000 ) ;
#2264=CARTESIAN_POINT ( 'NONE',  ( -41.99999999999996447, 60.00000000000002842, 23.64999999999999858 ) ) ;
#2270=CARTESIAN_POINT ( 'NONE',  ( 25.00000000000004263, -44.99999999999995737, 11.45643923738958314 ) ) ;
#2271=DIRECTION ( 'NONE',  ( 1.000000000000000000, -0.000000000000000000, -0.000000000000000000 ) ) ;
#2276=ORIENTED_EDGE ( 'NONE', *, *, #6083, .F. ) ;
#2283=DIRECTION ( 'NONE',  ( -1.000000000000000000, 0.000000000000000000, 0.000000000000000000 ) ) ;
#2284=CARTESIAN_POINT ( 'NONE',  ( -34.83673358847238433, -43.69081521296089221, 11.52653374317613810 ) ) ;
#2293=APPLICATION_CONTEXT ( 'automotive_design' ) ;
#2294=ORIENTED_EDGE ( 'NONE', *, *, #4818, .T. ) ;
#2295=CONICAL_SURFACE ( 'NONE', #8620, 1.649999999999998579, 1.029744258676653645 ) ;
#2318=VECTOR ( 'NONE', #5441, 1000.000000000000000 ) ;
#2319=DIRECTION ( 'NONE',  ( -0.000000000000000000, 1.000000000000000000, -0.000000000000000000 ) ) ;
#2329=CARTESIAN_POINT ( 'NONE',  ( 31.31030599380072488, -40.16344083911685914, 12.43538147425379492 ) ) ;
#2334=ORIENTED_EDGE ( 'NONE', *, *, #1974, .T. ) ;
#2342=CARTESIAN_POINT ( 'NONE',  ( -30.00000000000000000, -49.99999999999997158, 0.000000000000000000 ) ) ;
#2344=ORIENTED_EDGE ( 'NONE', *, *, #1018, .F. ) ;
#2348=EDGE_LOOP ( 'NONE', ( #6889, #2040, #6457 ) ) ;
#2349=ADVANCED_FACE ( 'NONE', ( #1623 ), #3574, .F. ) ;
#2354=AXIS2_PLACEMENT_3D ( 'NONE', #2982, #3512, #6476 ) ;
#2357=CONICAL_SURFACE ( 'NONE', #3061, 1.649999999999998579, 1.029744258676653645 ) ;
#2372=AXIS2_PLACEMENT_3D ( 'NONE', #7189, #358, #7108 ) ;
#2377=CARTESIAN_POINT ( 'NONE',  ( -26.69235372381821847, -48.76359959685383672, 12.05680772549333923 ) ) ;
#2379=EDGE_CURVE ( 'NONE', #8500, #6529, #6337, .T. ) ;
#2380=ORIENTED_EDGE ( 'NONE', *, *, #7605, .T. ) ;
#2388=CARTESIAN_POINT ( 'NONE',  ( -50.00000000000002842, -44.99999999999997158, -2.099999999999997868 ) ) ;
#2391=ORIENTED_EDGE ( 'NONE', *, *, #8234, .T. ) ;
#2395=EDGE_CURVE ( 'NONE', #1100, #724, #919, .T. ) ;
#2397=DIRECTION ( 'NONE',  ( -1.000000000000000000, -0.000000000000000000, -0.000000000000000000 ) ) ;
#2401=AXIS2_PLACEMENT_3D ( 'NONE', #5782, #433, #1024 ) ;
#2416=LINE ( 'NONE', #1081, #605 ) ;
#2419=CARTESIAN_POINT ( 'NONE',  ( -41.99999999999996447, 47.00857997860455129, 22.00000000000000000 ) ) ;
#2426=DIRECTION ( 'NONE',  ( -0.000000000000000000, -0.000000000000000000, -1.000000000000000000 ) ) ;
#2441=DIRECTION ( 'NONE',  ( 0.000000000000000000, 0.000000000000000000, -1.000000000000000000 ) ) ;
#2452=CARTESIAN_POINT ( 'NONE',  ( 25.00000000000003553, -45.33027059730881092, 11.45643923738957781 ) ) ;
#2454=LINE ( 'NONE', #7202, #2119 ) ;
#2462=ORIENTED_EDGE ( 'NONE', *, *, #395, .F. ) ;
#2464=CARTESIAN_POINT ( 'NONE',  ( -33.31087205654255712, -48.76061935842974293, 12.05589577412332680 ) ) ;
#2467=CARTESIAN_POINT ( 'NONE',  ( -41.99999999999996447, 48.00000000000002842, -22.00000000000000000 ) ) ;
#2472=EDGE_CURVE ( 'NONE', #1354, #5482, #2908, .T. ) ;
#2477=B_SPLINE_CURVE_WITH_KNOTS ( 'NONE', 3,
 ( #2199, #4884, #4218, #205, #2907, #5576, #8284, #1121, #992, #2377, #1614, #5052, #4303, #7742, #5011, #2991, #4968, #1705 ),
 .UNSPECIFIED., .F., .F.,
 ( 4, 2, 2, 2, 2, 2, 2, 2, 4 ),
 ( 0.02369462427231873447, 0.02468136329545929375, 0.02566810231859985303, 0.02665484134174040884, 0.02764158036488096812, 0.02862831938802152740, 0.02961505841116208321, 0.03060179743430264249, 0.03158853645744320177 ),
 .UNSPECIFIED. ) ;
#2481=ADVANCED_FACE ( 'NONE', ( #7752 ), #1049, .F. ) ;
#2486=VERTEX_POINT ( 'NONE', #7882 ) ;
#2492=CARTESIAN_POINT ( 'NONE',  ( 34.24325503137513493, -42.35030295949444934, 11.75814120956404629 ) ) ;
#2499=PRESENTATION_STYLE_ASSIGNMENT (( #8533 ) ) ;
#2509=CARTESIAN_POINT ( 'NONE',  ( -33.97303272786269446, -48.05319586029032308, 11.85336373935253285 ) ) ;
#2510=DIRECTION ( 'NONE',  ( -0.000000000000000000, 1.000000000000000000, -0.000000000000000000 ) ) ;
#2512=LINE ( 'NONE', #3660, #4539 ) ;
#2514=VERTEX_POINT ( 'NONE', #5897 ) ;
#2521=CARTESIAN_POINT ( 'NONE',  ( -41.99999999999996447, 48.00000000000002842, 23.64999999999999858 ) ) ;
#2533=CARTESIAN_POINT ( 'NONE',  ( -41.99999999999996447, 48.00000000000002842, -22.00000000000000000 ) ) ;
#2541=DIRECTION ( 'NONE',  ( -0.000000000000000000, 1.000000000000000000, -0.000000000000000000 ) ) ;
#2551=CARTESIAN_POINT ( 'NONE',  ( 30.66531197710604317, -49.96635986460696444, 12.48644052906005264 ) ) ;
#2553=ORIENTED_EDGE ( 'NONE', *, *, #3495, .F. ) ;
#2554=AXIS2_PLACEMENT_3D ( 'NONE', #7787, #1707, #3692 ) ;
#2557=EDGE_LOOP ( 'NONE', ( #3044, #8114, #7247, #3662 ) ) ;
#2569=VECTOR ( 'NONE', #3829, 1000.000000000000000 ) ;
#2576=ORIENTED_EDGE ( 'NONE', *, *, #1539, .T. ) ;
#2585=DIRECTION ( 'NONE',  ( 0.000000000000000000, 1.000000000000000000, 0.000000000000000000 ) ) ;
#2586=DIRECTION ( 'NONE',  ( 0.000000000000000000, 0.000000000000000000, 1.000000000000000000 ) ) ;
#2589=CARTESIAN_POINT ( 'NONE',  ( -30.00000000000000000, 60.00000000000002842, 12.49999999999998046 ) ) ;
#2594=VERTEX_POINT ( 'NONE', #7923 ) ;
#2596=SURFACE_STYLE_USAGE ( .BOTH. , #1344 ) ;
#2602=VERTEX_POINT ( 'NONE', #1889 ) ;
#2629=ORIENTED_EDGE ( 'NONE', *, *, #911, .F. ) ;
#2639=( NAMED_UNIT ( * ) PLANE_ANGLE_UNIT ( ) SI_UNIT ( $, .RADIAN. ) );
#2650=ORIENTED_EDGE ( 'NONE', *, *, #5685, .T. ) ;
#2657=ADVANCED_BREP_SHAPE_REPRESENTATION ( '', ( #2810, #2554 ), #5211 ) ;
#2661=CYLINDRICAL_SURFACE ( 'NONE', #4685, 4.999999999999969802 ) ;
#2663=ORIENTED_EDGE ( 'NONE', *, *, #2951, .F. ) ;
#2673=ORIENTED_EDGE ( 'NONE', *, *, #5647, .F. ) ;
#2679=EDGE_LOOP ( 'NONE', ( #7568, #1238, #5361, #8662 ) ) ;
#2682=CARTESIAN_POINT ( 'NONE',  ( -45.00000000000003553, -44.99999999999997158, 0.000000000000000000 ) ) ;
#2683=DIRECTION ( 'NONE',  ( 0.000000000000000000, 0.000000000000000000, 1.000000000000000000 ) ) ;
#2687=FACE_OUTER_BOUND ( 'NONE', #4096, .T. ) ;
#2688=ORIENTED_EDGE ( 'NONE', *, *, #4234, .T. ) ;
#2734=ORIENTED_EDGE ( 'NONE', *, *, #2094, .T. ) ;
#2744=VECTOR ( 'NONE', #2174, 1000.000000000000000 ) ;
#2749=CARTESIAN_POINT ( 'NONE',  ( 27.48332863331305731, -49.33273298888234848, 12.24717930254580267 ) ) ;
#2760=FACE_OUTER_BOUND ( 'NONE', #1152, .T. ) ;
#2769=VERTEX_POINT ( 'NONE', #5395 ) ;
#2771=EDGE_CURVE ( 'NONE', #2602, #3280, #4747, .T. ) ;
#2774=CARTESIAN_POINT ( 'NONE',  ( 42.00000000000000711, 48.00000000000002842, 20.34999999999992326 ) ) ;
#2776=CARTESIAN_POINT ( 'NONE',  ( -49.99999999999997158, -59.99999999999997158, 30.00000000000000000 ) ) ;
#2777=CARTESIAN_POINT ( 'NONE',  ( 42.00000000000000711, 48.00000000000002842, 21.99999999999992184 ) ) ;
#2798=CARTESIAN_POINT ( 'NONE',  ( 30.00000000000000000, -39.99999999999998579, 12.49999999999996625 ) ) ;
#2799=DIRECTION ( 'NONE',  ( -0.000000000000000000, -0.000000000000000000, 1.000000000000000000 ) ) ;
#2801=DIRECTION ( 'NONE',  ( 0.5150380749100560429, 1.049727191138617340E-16, 0.8571673007021112234 ) ) ;
#2810=MANIFOLD_SOLID_BREP ( 'Mirror1', #679 ) ;
#2830=AXIS2_PLACEMENT_3D ( 'NONE', #3421, #3331, #2143 ) ;
#2838=ORIENTED_EDGE ( 'NONE', *, *, #1692, .F. ) ;
#2842=CARTESIAN_POINT ( 'NONE',  ( 28.37719198635490869, -40.25948930238541124, 12.39794155511764373 ) ) ;
#2843=DIRECTION ( 'NONE',  ( 0.000000000000000000, 0.000000000000000000, -1.000000000000000000 ) ) ;
#2845=ADVANCED_FACE ( 'NONE', ( #2061 ), #4269, .F. ) ;
#2857=VECTOR ( 'NONE', #6022, 1000.000000000000000 ) ;
#2859=CARTESIAN_POINT ( 'NONE',  ( 42.00000000000000711, 60.00000000000002842, 23.64999999999992042 ) ) ;
#2863=EDGE_CURVE ( 'NONE', #207, #1713, #1165, .T. ) ;
#2867=AXIS2_PLACEMENT_3D ( 'NONE', #1051, #1005, #3743 ) ;
#2881=PRODUCT_DEFINITION ( 'UNKNOWN', '', #1724, #4236 ) ;
#2882=CARTESIAN_POINT ( 'NONE',  ( 30.00000000000000000, -49.99999999999997158, 12.49999999999995914 ) ) ;
#2889=CARTESIAN_POINT ( 'NONE',  ( -25.67300017005173274, -42.48926715326583547, 11.72748501658995579 ) ) ;
#2907=CARTESIAN_POINT ( 'NONE',  ( -25.25955351082667022, -46.62311395930105107, 11.56703930231305932 ) ) ;
#2908=CIRCLE ( 'NONE', #3320, 1.649999999999998579 ) ;
#2909=FACE_BOUND ( 'NONE', #766, .T. ) ;
#2915=CYLINDRICAL_SURFACE ( 'NONE', #5169, 12.49999999999998046 ) ;
#2920=EDGE_CURVE ( 'NONE', #6416, #8159, #7221, .T. ) ;
#2931=CARTESIAN_POINT ( 'NONE',  ( -41.99999999999996447, 48.00000000000002842, -20.35000000000000142 ) ) ;
#2951=EDGE_CURVE ( 'NONE', #1713, #207, #5673, .T. ) ;
#2961=DIRECTION ( 'NONE',  ( 0.000000000000000000, 0.000000000000000000, 1.000000000000000000 ) ) ;
#2964=VERTEX_POINT ( 'NONE', #5533 ) ;
#2969=DIRECTION ( 'NONE',  ( -0.000000000000000000, 1.000000000000000000, -0.000000000000000000 ) ) ;
#2975=CARTESIAN_POINT ( 'NONE',  ( -45.00000000000003553, -44.99999999999997158, 0.000000000000000000 ) ) ;
#2982=CARTESIAN_POINT ( 'NONE',  ( 42.00000000000000711, 60.00000000000002842, 21.99999999999992184 ) ) ;
#2991=CARTESIAN_POINT ( 'NONE',  ( -29.33468802289397104, -49.96635986460699286, 12.48644052906006685 ) ) ;
#2998=EDGE_CURVE ( 'NONE', #1128, #5614, #2153, .T. ) ;
#3000=ORIENTED_EDGE ( 'NONE', *, *, #3495, .T. ) ;
#3014=DIRECTION ( 'NONE',  ( 1.000000000000000000, -0.000000000000000000, -0.000000000000000000 ) ) ;
#3019=EDGE_CURVE ( 'NONE', #58, #3140, #4277, .T. ) ;
#3025=LINE ( 'NONE', #1740, #1699 ) ;
#3044=ORIENTED_EDGE ( 'NONE', *, *, #4327, .F. ) ;
#3057=DIRECTION ( 'NONE',  ( -0.000000000000000000, 1.000000000000000000, -0.000000000000000000 ) ) ;
#3061=AXIS2_PLACEMENT_3D ( 'NONE', #6113, #4264, #6816 ) ;
#3068=CIRCLE ( 'NONE', #7984, 1.649999999999998579 ) ;
#3075=CARTESIAN_POINT ( 'NONE',  ( 32.51929462645154700, -40.66893875716690587, 12.24660140962717136 ) ) ;
#3081=ORIENTED_EDGE ( 'NONE', *, *, #5478, .F. ) ;
#3084=ORIENTED_EDGE ( 'NONE', *, *, #995, .F. ) ;
#3088=DIRECTION ( 'NONE',  ( 1.049727191138618079E-16, 0.5150380749100549327, -0.8571673007021118895 ) ) ;
#3103=CARTESIAN_POINT ( 'NONE',  ( -30.00000000000000000, -49.99999999999997158, 12.49999999999997335 ) ) ;
#3122=CARTESIAN_POINT ( 'NONE',  ( -49.99999999999997158, -59.99999999999997158, 30.00000000000000000 ) ) ;
#3126=EDGE_CURVE ( 'NONE', #8149, #8159, #451, .T. ) ;
#3130=DIRECTION ( 'NONE',  ( 0.000000000000000000, 0.000000000000000000, 1.000000000000000000 ) ) ;
#3131=EDGE_CURVE ( 'NONE', #1305, #2514, #6801, .T. ) ;
#3140=VERTEX_POINT ( 'NONE', #1796 ) ;
#3149=( GEOMETRIC_REPRESENTATION_CONTEXT ( 3 ) GLOBAL_UNCERTAINTY_ASSIGNED_CONTEXT ( ( #90 ) ) GLOBAL_UNIT_ASSIGNED_CONTEXT ( ( #727, #2639, #3344 ) ) REPRESENTATION_CONTEXT ( 'NONE', 'WORKASPACE' ) );
#3156=ORIENTED_EDGE ( 'NONE', *, *, #4757, .T. ) ;
#3162=CARTESIAN_POINT ( 'NONE',  ( 30.65872425187075123, -40.04081516742414948, 12.48372095990569797 ) ) ;
#3165=DIRECTION ( 'NONE',  ( 0.000000000000000000, 0.000000000000000000, 1.000000000000000000 ) ) ;
#3168=VERTEX_POINT ( 'NONE', #2419 ) ;
#3173=CARTESIAN_POINT ( 'NONE',  ( -31.30653513488008244, -49.83744928702515864, 12.43572992548471845 ) ) ;
#3181=EDGE_CURVE ( 'NONE', #6859, #6385, #3292, .T. ) ;
#3186=CARTESIAN_POINT ( 'NONE',  ( 50.00000000000002842, -44.99999999999997158, 0.000000000000000000 ) ) ;
#3187=AXIS2_PLACEMENT_3D ( 'NONE', #5490, #7607, #8198 ) ;
#3189=CARTESIAN_POINT ( 'NONE',  ( -30.00000000000000000, -45.00000000000000000, -30.00100000000000122 ) ) ;
#3196=ADVANCED_FACE ( 'NONE', ( #7958, #7916 ), #5140, .F. ) ;
#3199=CARTESIAN_POINT ( 'NONE',  ( 45.00000000000003553, -44.99999999999997158, 0.000000000000000000 ) ) ;
#3206=CIRCLE ( 'NONE', #4048, 1.649999999999998579 ) ;
#3215=EDGE_CURVE ( 'NONE', #6557, #8668, #1881, .T. ) ;
#3218=ORIENTED_EDGE ( 'NONE', *, *, #3900, .T. ) ;
#3219=AXIS2_PLACEMENT_3D ( 'NONE', #3186, #7766, #2441 ) ;
#3228=DIRECTION ( 'NONE',  ( 1.049727191138618079E-16, 0.5150380749100549327, -0.8571673007021118895 ) ) ;
#3231=DIRECTION ( 'NONE',  ( 0.000000000000000000, 0.000000000000000000, 1.000000000000000000 ) ) ;
#3244=DIRECTION ( 'NONE',  ( 0.000000000000000000, 0.000000000000000000, 1.000000000000000000 ) ) ;
#3248=ORIENTED_EDGE ( 'NONE', *, *, #5233, .T. ) ;
#3257=CARTESIAN_POINT ( 'NONE',  ( 31.62245743458239033, -49.74093594125425000, 12.39808714042238869 ) ) ;
#3260=CIRCLE ( 'NONE', #7612, 1.649999999999998579 ) ;
#3280=VERTEX_POINT ( 'NONE', #6716 ) ;
#3285=VECTOR ( 'NONE', #6679, 1000.000000000000000 ) ;
#3292=CIRCLE ( 'NONE', #8224, 12.49999999999997335 ) ;
#3296=EDGE_LOOP ( 'NONE', ( #4294, #8539, #5437, #5285 ) ) ;
#3301=ORIENTED_EDGE ( 'NONE', *, *, #4573, .T. ) ;
#3303=CARTESIAN_POINT ( 'NONE',  ( 30.00000000000000000, 60.00000000000002842, 12.49999999999996625 ) ) ;
#3306=CARTESIAN_POINT ( 'NONE',  ( 34.99999999999998579, -45.32948160161797091, 11.45643923738956893 ) ) ;
#3309=VERTEX_POINT ( 'NONE', #8185 ) ;
#3312=ORIENTED_EDGE ( 'NONE', *, *, #3126, .T. ) ;
#3320=AXIS2_PLACEMENT_3D ( 'NONE', #5224, #2510, #3872 ) ;
#3323=EDGE_CURVE ( 'NONE', #6288, #6845, #674, .T. ) ;
#3331=DIRECTION ( 'NONE',  ( -0.000000000000000000, 1.000000000000000000, -0.000000000000000000 ) ) ;
#3332=FACE_OUTER_BOUND ( 'NONE', #567, .T. ) ;
#3340=VECTOR ( 'NONE', #7589, 1000.000000000000000 ) ;
#3341=ORIENTED_EDGE ( 'NONE', *, *, #2103, .F. ) ;
#3344=( NAMED_UNIT ( * ) SI_UNIT ( $, .STERADIAN. ) SOLID_ANGLE_UNIT ( ) );
#3354=VECTOR ( 'NONE', #8380, 1000.000000000000000 ) ;
#3368=EDGE_LOOP ( 'NONE', ( #3693, #8359, #249, #3301 ) ) ;
#3375=EDGE_CURVE ( 'NONE', #912, #2594, #6672, .T. ) ;
#3392=CARTESIAN_POINT ( 'NONE',  ( 50.00000000000002842, 60.00000000000002842, 30.00000000000000000 ) ) ;
#3421=CARTESIAN_POINT ( 'NONE',  ( 42.00000000000000711, 60.00000000000002842, 21.99999999999992184 ) ) ;
#3424=CONICAL_SURFACE ( 'NONE', #7921, 1.649999999999998579, 1.029744258676653645 ) ;
#3430=ORIENTED_EDGE ( 'NONE', *, *, #3749, .F. ) ;
#3445=AXIS2_PLACEMENT_3D ( 'NONE', #534, #4645, #3244 ) ;
#3462=LINE ( 'NONE', #6184, #3753 ) ;
#3464=LINE ( 'NONE', #6145, #5777 ) ;
#3475=ORIENTED_EDGE ( 'NONE', *, *, #395, .T. ) ;
#3477=CARTESIAN_POINT ( 'NONE',  ( -31.31024842726172608, -40.16330870357086980, 12.43543189630224077 ) ) ;
#3482=VECTOR ( 'NONE', #4649, 1000.000000000000000 ) ;
#3495=EDGE_CURVE ( 'NONE', #7164, #6529, #645, .T. ) ;
#3505=EDGE_CURVE ( 'NONE', #4829, #1713, #151, .T. ) ;
#3506=CARTESIAN_POINT ( 'NONE',  ( -26.69211319910860070, -41.23645700522185820, 12.05676622698253730 ) ) ;
#3512=DIRECTION ( 'NONE',  ( -0.000000000000000000, 1.000000000000000000, -0.000000000000000000 ) ) ;
#3513=EDGE_LOOP ( 'NONE', ( #7235, #1382 ) ) ;
#3520=DIRECTION ( 'NONE',  ( 1.049727191138618079E-16, 0.5150380749100549327, -0.8571673007021118895 ) ) ;
#3523=DIRECTION ( 'NONE',  ( -0.000000000000000000, 1.000000000000000000, -0.000000000000000000 ) ) ;
#3529=AXIS2_PLACEMENT_3D ( 'NONE', #2975, #4460, #3799 ) ;
#3541=DIRECTION ( 'NONE',  ( 0.000000000000000000, 0.000000000000000000, 1.000000000000000000 ) ) ;
#3545=CARTESIAN_POINT ( 'NONE',  ( 27.34989276402963299, -40.75696118185767602, 12.21663313815757590 ) ) ;
#3550=ORIENTED_EDGE ( 'NONE', *, *, #3019, .T. ) ;
#3551=DIRECTION ( 'NONE',  ( -0.000000000000000000, 1.000000000000000000, -0.000000000000000000 ) ) ;
#3562=CARTESIAN_POINT ( 'NONE',  ( -33.05528180196482424, -41.02872310104125830, 12.12402686769023852 ) ) ;
#3571=EDGE_LOOP ( 'NONE', ( #6107, #236, #6486 ) ) ;
#3573=CARTESIAN_POINT ( 'NONE',  ( -30.00000000000000000, -49.99999999999997158, 0.000000000000000000 ) ) ;
#3574=CYLINDRICAL_SURFACE ( 'NONE', #7398, 1.649999999999998579 ) ;
#3584=CARTESIAN_POINT ( 'NONE',  ( -30.00000000000000000, -40.00000000000002132, 12.49999999999998046 ) ) ;
#3589=CARTESIAN_POINT ( 'NONE',  ( 25.66790131137006625, -42.48249851487847906, 11.72687238757475114 ) ) ;
#3602=CARTESIAN_POINT ( 'NONE',  ( -30.00000000000000000, -40.00000000000002132, 12.49999999999998046 ) ) ;
#3607=ORIENTED_EDGE ( 'NONE', *, *, #2863, .F. ) ;
#3610=EDGE_LOOP ( 'NONE', ( #6790, #5894, #4783 ) ) ;
#3611=CIRCLE ( 'NONE', #5858, 12.49999999999998757 ) ;
#3615=ADVANCED_FACE ( 'NONE', ( #6888 ), #429, .F. ) ;
#3617=CARTESIAN_POINT ( 'NONE',  ( 42.00000000000000711, 48.00000000000002842, 21.99999999999992184 ) ) ;
#3625=VECTOR ( 'NONE', #3520, 1000.000000000000000 ) ;
#3637=CARTESIAN_POINT ( 'NONE',  ( 42.00000000000000711, 48.00000000000002842, -21.99999999999992184 ) ) ;
#3638=ORIENTED_EDGE ( 'NONE', *, *, #5580, .F. ) ;
#3644=DIRECTION ( 'NONE',  ( -0.000000000000000000, 1.000000000000000000, -0.000000000000000000 ) ) ;
#3657=CARTESIAN_POINT ( 'NONE',  ( 42.00000000000000711, 60.00000000000002842, -21.99999999999992184 ) ) ;
#3659=EDGE_CURVE ( 'NONE', #6288, #6070, #6934, .T. ) ;
#3660=CARTESIAN_POINT ( 'NONE',  ( -41.99999999999996447, 48.00000000000002842, -20.35000000000000142 ) ) ;
#3662=ORIENTED_EDGE ( 'NONE', *, *, #2998, .F. ) ;
#3668=AXIS2_PLACEMENT_3D ( 'NONE', #4561, #991, #3165 ) ;
#3679=ADVANCED_FACE ( 'NONE', ( #1815 ), #5564, .F. ) ;
#3690=CARTESIAN_POINT ( 'NONE',  ( 30.00000000000000000, -49.99999999999997158, -1.102182119232617753E-14 ) ) ;
#3692=DIRECTION ( 'NONE',  ( 1.000000000000000000, 0.000000000000000000, 0.000000000000000000 ) ) ;
#3693=ORIENTED_EDGE ( 'NONE', *, *, #5860, .F. ) ;
#3696=VECTOR ( 'NONE', #2426, 1000.000000000000000 ) ;
#3712=CARTESIAN_POINT ( 'NONE',  ( 30.00000000000000000, 60.00000000000002842, -1.102182119232617753E-14 ) ) ;
#3729=CARTESIAN_POINT ( 'NONE',  ( 25.12952813221809123, -46.14268964625811265, 11.51215629180720512 ) ) ;
#3732=CYLINDRICAL_SURFACE ( 'NONE', #7375, 2.099999999999997868 ) ;
#3743=DIRECTION ( 'NONE',  ( 0.000000000000000000, 0.000000000000000000, 1.000000000000000000 ) ) ;
#3749=EDGE_CURVE ( 'NONE', #1695, #5699, #5282, .T. ) ;
#3752=CARTESIAN_POINT ( 'NONE',  ( 30.00000000000000000, -49.99999999999997158, -1.102182119232617753E-14 ) ) ;
#3753=VECTOR ( 'NONE', #6927, 1000.000000000000000 ) ;
#3755=EDGE_CURVE ( 'NONE', #2964, #4084, #3462, .T. ) ;
#3760=ADVANCED_FACE ( 'NONE', ( #759 ), #5859, .F. ) ;
#3762=AXIS2_PLACEMENT_3D ( 'NONE', #2533, #7241, #5336 ) ;
#3769=EDGE_CURVE ( 'NONE', #3168, #6235, #4952, .T. ) ;
#3772=CARTESIAN_POINT ( 'NONE',  ( 30.00000000000000000, -39.99999999999998579, 12.49999999999996625 ) ) ;
#3775=DIRECTION ( 'NONE',  ( -1.000000000000000000, -0.000000000000000000, -0.000000000000000000 ) ) ;
#3777=EDGE_CURVE ( 'NONE', #2594, #724, #2068, .T. ) ;
#3780=CARTESIAN_POINT ( 'NONE',  ( -30.00000000000000000, -49.99999999999997158, 0.000000000000000000 ) ) ;
#3793=ORIENTED_EDGE ( 'NONE', *, *, #8340, .T. ) ;
#3796=DIRECTION ( 'NONE',  ( -0.000000000000000000, -0.000000000000000000, -1.000000000000000000 ) ) ;
#3799=DIRECTION ( 'NONE',  ( 0.000000000000000000, 0.000000000000000000, 1.000000000000000000 ) ) ;
#3800=ADVANCED_FACE ( 'NONE', ( #1509 ), #4887, .F. ) ;
#3810=CARTESIAN_POINT ( 'NONE',  ( 25.17038609909130287, -46.30459253935128316, 11.52942094433410070 ) ) ;
#3815=DIRECTION ( 'NONE',  ( 0.000000000000000000, 0.000000000000000000, -1.000000000000000000 ) ) ;
#3821=COLOUR_RGB ( '', 0.66274510, 0.83137255, 0.94901961) ;
#3822=ADVANCED_FACE ( 'NONE', ( #1422 ), #4117, .F. ) ;
#3829=DIRECTION ( 'NONE',  ( -0.000000000000000000, 1.000000000000000000, -0.000000000000000000 ) ) ;
#3844=FACE_OUTER_BOUND ( 'NONE', #150, .T. ) ;
#3859=DIRECTION ( 'NONE',  ( -0.000000000000000000, 1.000000000000000000, -0.000000000000000000 ) ) ;
#3863=DIRECTION ( 'NONE',  ( 1.000000000000000000, 0.000000000000000000, 0.000000000000000000 ) ) ;
#3865=AXIS2_PLACEMENT_3D ( 'NONE', #45, #5417, #3541 ) ;
#3868=EDGE_LOOP ( 'NONE', ( #8156, #5342 ) ) ;
#3869=ORIENTED_EDGE ( 'NONE', *, *, #3181, .T. ) ;
#3871=CARTESIAN_POINT ( 'NONE',  ( -34.67778767197271605, -46.77334385938317496, 11.59192968702633486 ) ) ;
#3872=DIRECTION ( 'NONE',  ( 0.000000000000000000, 0.000000000000000000, 1.000000000000000000 ) ) ;
#3874=CARTESIAN_POINT ( 'NONE',  ( 32.23131546658671454, -49.48665499171476512, 12.30309571437651428 ) ) ;
#3887=CARTESIAN_POINT ( 'NONE',  ( 29.66573552397922242, -49.99999999999991473, 12.49999999999996803 ) ) ;
#3888=VECTOR ( 'NONE', #4293, 1000.000000000000000 ) ;
#3889=DIRECTION ( 'NONE',  ( -0.000000000000000000, -0.000000000000000000, 1.000000000000000000 ) ) ;
#3900=EDGE_CURVE ( 'NONE', #5916, #2514, #4777, .T. ) ;
#3902=FACE_OUTER_BOUND ( 'NONE', #8146, .T. ) ;
#3911=ORIENTED_EDGE ( 'NONE', *, *, #778, .F. ) ;
#3917=DIRECTION ( 'NONE',  ( 1.000000000000000000, -0.000000000000000000, -0.000000000000000000 ) ) ;
#3921=EDGE_CURVE ( 'NONE', #5699, #1695, #4793, .T. ) ;
#3935=CARTESIAN_POINT ( 'NONE',  ( 50.00000000000002842, -44.99999999999997158, -2.099999999999997868 ) ) ;
#3939=DIRECTION ( 'NONE',  ( -0.000000000000000000, 1.000000000000000000, -0.000000000000000000 ) ) ;
#3952=ORIENTED_EDGE ( 'NONE', *, *, #7252, .F. ) ;
#3955=DIRECTION ( 'NONE',  ( 0.000000000000000000, 0.000000000000000000, 1.000000000000000000 ) ) ;
#3984=CARTESIAN_POINT ( 'NONE',  ( -41.99999999999996447, 60.00000000000002842, 23.64999999999999858 ) ) ;
#3988=DIRECTION ( 'NONE',  ( 0.000000000000000000, 0.000000000000000000, 1.000000000000000000 ) ) ;
#3999=FILL_AREA_STYLE ('',( #637 ) ) ;
#4002=CARTESIAN_POINT ( 'NONE',  ( 34.33292552453226421, -47.51618826727536771, 11.72657454140205679 ) ) ;
#4005=ORIENTED_EDGE ( 'NONE', *, *, #3131, .T. ) ;
#4016=ADVANCED_FACE ( 'NONE', ( #4995 ), #4422, .F. ) ;
#4018=VECTOR ( 'NONE', #7571, 1000.000000000000000 ) ;
#4022=ADVANCED_FACE ( 'NONE', ( #1738 ), #7315, .F. ) ;
#4029=EDGE_CURVE ( 'NONE', #1100, #912, #4225, .T. ) ;
#4030=CARTESIAN_POINT ( 'NONE',  ( 42.00000000000000711, 60.00000000000002842, 21.99999999999992184 ) ) ;
#4035=VERTEX_POINT ( 'NONE', #1688 ) ;
#4044=CARTESIAN_POINT ( 'NONE',  ( -41.99999999999996447, 60.00000000000002842, -20.35000000000000142 ) ) ;
#4048=AXIS2_PLACEMENT_3D ( 'NONE', #7300, #1257, #3955 ) ;
#4050=VECTOR ( 'NONE', #708, 1000.000000000000000 ) ;
#4053=EDGE_LOOP ( 'NONE', ( #4399, #5222, #3952, #6276 ) ) ;
#4055=ADVANCED_FACE ( 'NONE', ( #8478 ), #5481, .F. ) ;
#4064=UNCERTAINTY_MEASURE_WITH_UNIT (LENGTH_MEASURE( 1.000000000000000082E-05 ), #7121, 'distance_accuracy_value', 'NONE');
#4084=VERTEX_POINT ( 'NONE', #7728 ) ;
#4088=AXIS2_PLACEMENT_3D ( 'NONE', #4287, #8136, #2095 ) ;
#4091=FACE_BOUND ( 'NONE', #6510, .T. ) ;
#4092=ORIENTED_EDGE ( 'NONE', *, *, #1008, .F. ) ;
#4093=ADVANCED_FACE ( 'NONE', ( #4378 ), #8517, .F. ) ;
#4096=EDGE_LOOP ( 'NONE', ( #1529, #3156, #424 ) ) ;
#4097=ORIENTED_EDGE ( 'NONE', *, *, #3505, .T. ) ;
#4108=CARTESIAN_POINT ( 'NONE',  ( 26.02696727213731265, -48.05319586029025913, 11.85336373935252041 ) ) ;
#4117=CYLINDRICAL_SURFACE ( 'NONE', #6982, 4.999999999999969802 ) ;
#4132=CARTESIAN_POINT ( 'NONE',  ( -45.00000000000003553, -44.99999999999997158, -2.099999999999997868 ) ) ;
#4134=CARTESIAN_POINT ( 'NONE',  ( 34.99999999999998579, -44.99999999999995737, -30.00100000000000122 ) ) ;
#4135=FACE_BOUND ( 'NONE', #1401, .T. ) ;
#4139=EDGE_CURVE ( 'NONE', #912, #1100, #5772, .T. ) ;
#4156=CARTESIAN_POINT ( 'NONE',  ( -49.99999999999997158, -59.99999999999997158, 30.00000000000000000 ) ) ;
#4159=CARTESIAN_POINT ( 'NONE',  ( -28.68969400619928578, -40.16344083911688045, 12.43538147425380203 ) ) ;
#4164=EDGE_LOOP ( 'NONE', ( #1253, #7509, #7297, #5167 ) ) ;
#4166=ORIENTED_EDGE ( 'NONE', *, *, #7092, .F. ) ;
#4173=CARTESIAN_POINT ( 'NONE',  ( 50.00000000000002842, 60.00000000000002842, -30.00000000000000000 ) ) ;
#4176=FACE_OUTER_BOUND ( 'NONE', #4607, .T. ) ;
#4178=AXIS2_PLACEMENT_3D ( 'NONE', #4496, #6189, #5524 ) ;
#4185=ADVANCED_FACE ( 'NONE', ( #6453 ), #699, .F. ) ;
#4201=CARTESIAN_POINT ( 'NONE',  ( 26.94471819803519708, -41.02872310104123699, 12.12402686769023141 ) ) ;
#4205=CARTESIAN_POINT ( 'NONE',  ( 42.00000000000000711, 60.00000000000002842, -21.99999999999992184 ) ) ;
#4215=DIRECTION ( 'NONE',  ( 0.000000000000000000, 0.000000000000000000, 1.000000000000000000 ) ) ;
#4216=CARTESIAN_POINT ( 'NONE',  ( -33.76204298352917732, -41.69067313909257422, 11.92283337402248300 ) ) ;
#4218=CARTESIAN_POINT ( 'NONE',  ( -25.03224621535701289, -45.65699184524256538, 11.47067790983491875 ) ) ;
#4219=FACE_BOUND ( 'NONE', #6629, .T. ) ;
#4225=CIRCLE ( 'NONE', #3529, 2.099999999999997868 ) ;
#4226=DIRECTION ( 'NONE',  ( -0.000000000000000000, 1.000000000000000000, -0.000000000000000000 ) ) ;
#4234=EDGE_CURVE ( 'NONE', #8538, #6235, #6748, .T. ) ;
#4236=PRODUCT_DEFINITION_CONTEXT ( 'detailed design', #6332, 'design' ) ;
#4241=DIRECTION ( 'NONE',  ( -1.000000000000000000, 0.000000000000000000, -0.000000000000000000 ) ) ;
#4243=CARTESIAN_POINT ( 'NONE',  ( -27.77183716021333382, -40.51193879865776637, 12.30361675895773210 ) ) ;
#4261=CARTESIAN_POINT ( 'NONE',  ( -32.65010723597040254, -40.75696118185769734, 12.21663313815758478 ) ) ;
#4264=DIRECTION ( 'NONE',  ( -0.000000000000000000, 1.000000000000000000, -0.000000000000000000 ) ) ;
#4269=CONICAL_SURFACE ( 'NONE', #5526, 2.099999999999997868, 1.029744258676652313 ) ;
#4272=LINE ( 'NONE', #7485, #1089 ) ;
#4276=EDGE_LOOP ( 'NONE', ( #1927, #4092, #2391, #2334 ) ) ;
#4277=CIRCLE ( 'NONE', #454, 4.999999999999973355 ) ;
#4282=CARTESIAN_POINT ( 'NONE',  ( -45.00000000000003553, -44.99999999999997158, 0.000000000000000000 ) ) ;
#4284=DIRECTION ( 'NONE',  ( 0.000000000000000000, 0.000000000000000000, -1.000000000000000000 ) ) ;
#4286=CARTESIAN_POINT ( 'NONE',  ( 27.77933658956289520, -40.51720970344479866, 12.30204028087673152 ) ) ;
#4287=CARTESIAN_POINT ( 'NONE',  ( 50.00000000000002842, -44.99999999999997158, 0.000000000000000000 ) ) ;
#4293=DIRECTION ( 'NONE',  ( -0.000000000000000000, -0.000000000000000000, 1.000000000000000000 ) ) ;
#4294=ORIENTED_EDGE ( 'NONE', *, *, #4234, .F. ) ;
#4301=CARTESIAN_POINT ( 'NONE',  ( -30.32897932148009801, -40.00000000000001421, 12.49999999999998046 ) ) ;
#4303=CARTESIAN_POINT ( 'NONE',  ( -27.76868453341328546, -49.48665499171480775, 12.30309571437652671 ) ) ;
#4306=EDGE_CURVE ( 'NONE', #7279, #58, #2454, .T. ) ;
#4327=EDGE_CURVE ( 'NONE', #6070, #1128, #4693, .T. ) ;
#4335=DIRECTION ( 'NONE',  ( 0.000000000000000000, 0.000000000000000000, 1.000000000000000000 ) ) ;
#4337=CARTESIAN_POINT ( 'NONE',  ( 45.00000000000003553, -44.99999999999997158, 2.099999999999997868 ) ) ;
#4339=VECTOR ( 'NONE', #3228, 1000.000000000000000 ) ;
#4360=CARTESIAN_POINT ( 'NONE',  ( -34.33694741576523768, -47.50955795526805048, 11.72510588894414596 ) ) ;
#4362=DIRECTION ( 'NONE',  ( -0.000000000000000000, 1.000000000000000000, -0.000000000000000000 ) ) ;
#4363=PLANE ( 'NONE',  #2867 ) ;
#4365=EDGE_LOOP ( 'NONE', ( #7539, #4097, #5986, #7889, #5674 ) ) ;
#4377=CARTESIAN_POINT ( 'NONE',  ( -25.00000000000002487, -45.00000000000000000, 11.45643923738959025 ) ) ;
#4378=FACE_OUTER_BOUND ( 'NONE', #5762, .T. ) ;
#4392=CARTESIAN_POINT ( 'NONE',  ( -30.00000000000000000, -49.99999999999997158, 0.000000000000000000 ) ) ;
#4399=ORIENTED_EDGE ( 'NONE', *, *, #99, .T. ) ;
#4414=AXIS2_PLACEMENT_3D ( 'NONE', #3122, #3863, #6541 ) ;
#4422=CYLINDRICAL_SURFACE ( 'NONE', #2401, 1.649999999999998579 ) ;
#4425=DIRECTION ( 'NONE',  ( -0.000000000000000000, -0.000000000000000000, -1.000000000000000000 ) ) ;
#4428=EDGE_LOOP ( 'NONE', ( #1173, #210, #7022, #6852 ) ) ;
#4436=CARTESIAN_POINT ( 'NONE',  ( 45.00000000000003553, -44.99999999999997158, 0.000000000000000000 ) ) ;
#4438=SURFACE_STYLE_FILL_AREA ( #5138 ) ;
#4440=DIRECTION ( 'NONE',  ( -0.000000000000000000, 1.000000000000000000, -0.000000000000000000 ) ) ;
#4443=ORIENTED_EDGE ( 'NONE', *, *, #778, .T. ) ;
#4447=LINE ( 'NONE', #1806, #7068 ) ;
#4459=FACE_OUTER_BOUND ( 'NONE', #4551, .T. ) ;
#4460=DIRECTION ( 'NONE',  ( -1.000000000000000000, -0.000000000000000000, -0.000000000000000000 ) ) ;
#4462=FACE_OUTER_BOUND ( 'NONE', #7253, .T. ) ;
#4477=SHAPE_REPRESENTATION_RELATIONSHIP ( 'NONE' , 'NONE' ,  #6809, #2657 ) ;
#4495=CARTESIAN_POINT ( 'NONE',  ( -41.99999999999996447, 60.00000000000002842, -22.00000000000000000 ) ) ;
#4496=CARTESIAN_POINT ( 'NONE',  ( -49.99999999999997158, -59.99999999999997158, 30.00000000000000000 ) ) ;
#4512=CARTESIAN_POINT ( 'NONE',  ( 34.48171389889316885, -42.77717578641264140, 11.66923617342547992 ) ) ;
#4518=( NAMED_UNIT ( * ) PLANE_ANGLE_UNIT ( ) SI_UNIT ( $, .RADIAN. ) );
#4521=ADVANCED_FACE ( 'NONE', ( #8041 ), #6054, .F. ) ;
#4528=CARTESIAN_POINT ( 'NONE',  ( -34.87047186778190877, -46.14268964625814817, 11.51215629180721400 ) ) ;
#4532=DIRECTION ( 'NONE',  ( -0.000000000000000000, 1.000000000000000000, -0.000000000000000000 ) ) ;
#4534=ORIENTED_EDGE ( 'NONE', *, *, #6083, .T. ) ;
#4537=EDGE_LOOP ( 'NONE', ( #3475, #2135, #3550, #1501, #7473 ) ) ;
#4539=VECTOR ( 'NONE', #7840, 1000.000000000000000 ) ;
#4547=CARTESIAN_POINT ( 'NONE',  ( 30.00000000000001421, -49.99999999999997158, 12.49999999999995914 ) ) ;
#4548=DIRECTION ( 'NONE',  ( 1.000000000000000000, 0.000000000000000000, 0.000000000000000000 ) ) ;
#4551=EDGE_LOOP ( 'NONE', ( #337, #8326, #414, #7732 ) ) ;
#4556=AXIS2_PLACEMENT_3D ( 'NONE', #8699, #6620, #7289 ) ;
#4561=CARTESIAN_POINT ( 'NONE',  ( -41.99999999999996447, 48.00000000000002842, 22.00000000000000000 ) ) ;
#4566=CARTESIAN_POINT ( 'NONE',  ( 42.00000000000000711, 48.00000000000002842, 23.64999999999992042 ) ) ;
#4573=EDGE_CURVE ( 'NONE', #1053, #8058, #1548, .T. ) ;
#4578=DIRECTION ( 'NONE',  ( 0.000000000000000000, 0.000000000000000000, -1.000000000000000000 ) ) ;
#4607=EDGE_LOOP ( 'NONE', ( #1809, #8701, #6628, #1725 ) ) ;
#4615=DIRECTION ( 'NONE',  ( -1.000000000000000000, -0.000000000000000000, -0.000000000000000000 ) ) ;
#4623=VERTEX_POINT ( 'NONE', #104 ) ;
#4624=CARTESIAN_POINT ( 'NONE',  ( -30.00000000000000000, 60.00000000000002842, -12.49999999999998046 ) ) ;
#4628=DIRECTION ( 'NONE',  ( -0.000000000000000000, 1.000000000000000000, -0.000000000000000000 ) ) ;
#4635=VERTEX_POINT ( 'NONE', #8310 ) ;
#4645=DIRECTION ( 'NONE',  ( -0.000000000000000000, 1.000000000000000000, -0.000000000000000000 ) ) ;
#4649=DIRECTION ( 'NONE',  ( 0.000000000000000000, 1.000000000000000000, 0.000000000000000000 ) ) ;
#4653=AXIS2_PLACEMENT_3D ( 'NONE', #4495, #4628, #1142 ) ;
#4685=AXIS2_PLACEMENT_3D ( 'NONE', #7276, #3889, #4548 ) ;
#4690=CARTESIAN_POINT ( 'NONE',  ( -41.99999999999996447, 60.00000000000002842, 22.00000000000000000 ) ) ;
#4693=LINE ( 'NONE', #5429, #7033 ) ;
#4709=CARTESIAN_POINT ( 'NONE',  ( 33.05403370888239323, -48.97208017019577397, 12.12430375744700406 ) ) ;
#4732=AXIS2_PLACEMENT_3D ( 'NONE', #7926, #3917, #4578 ) ;
#4744=ORIENTED_EDGE ( 'NONE', *, *, #2472, .F. ) ;
#4747=LINE ( 'NONE', #3303, #3285 ) ;
#4753=ORIENTED_EDGE ( 'NONE', *, *, #4849, .F. ) ;
#4757=EDGE_CURVE ( 'NONE', #2964, #4999, #3464, .T. ) ;
#4769=CARTESIAN_POINT ( 'NONE',  ( 26.94219849796044031, -48.96939036817694557, 12.12340239416034748 ) ) ;
#4772=ORIENTED_EDGE ( 'NONE', *, *, #6650, .F. ) ;
#4776=CARTESIAN_POINT ( 'NONE',  ( -27.48070537354846365, -40.66893875716694140, 12.24660140962718735 ) ) ;
#4777=LINE ( 'NONE', #8178, #2263 ) ;
#4783=ORIENTED_EDGE ( 'NONE', *, *, #1008, .T. ) ;
#4793=CIRCLE ( 'NONE', #4088, 2.099999999999997868 ) ;
#4796=FACE_BOUND ( 'NONE', #3868, .T. ) ;
#4805=AXIS2_PLACEMENT_3D ( 'NONE', #313, #3014, #8391 ) ;
#4814=LINE ( 'NONE', #2882, #2744 ) ;
#4818=EDGE_CURVE ( 'NONE', #3280, #5819, #4939, .T. ) ;
#4821=AXIS2_PLACEMENT_3D ( 'NONE', #140, #4284, #4241 ) ;
#4823=CARTESIAN_POINT ( 'NONE',  ( -41.99999999999996447, 48.00000000000002842, 22.00000000000000000 ) ) ;
#4829=VERTEX_POINT ( 'NONE', #8399 ) ;
#4832=CONICAL_SURFACE ( 'NONE', #5593, 12.49999999999997335, 1.029744258676651869 ) ;
#4839=CARTESIAN_POINT ( 'NONE',  ( -49.99999999999997158, 60.00000000000002842, -30.00000000000000000 ) ) ;
#4840=CARTESIAN_POINT ( 'NONE',  ( -34.99999999999997868, -44.66998333124467280, 11.45643923738958847 ) ) ;
#4843=FACE_BOUND ( 'NONE', #3513, .T. ) ;
#4849=EDGE_CURVE ( 'NONE', #2769, #5614, #3025, .T. ) ;
#4856=ADVANCED_FACE ( 'NONE', ( #5744 ), #383, .F. ) ;
#4859=UNCERTAINTY_MEASURE_WITH_UNIT (LENGTH_MEASURE( 1.000000000000000082E-05 ), #372, 'distance_accuracy_value', 'NONE');
#4863=SHAPE_DEFINITION_REPRESENTATION ( #5709, #6809 ) ;
#4869=CARTESIAN_POINT ( 'NONE',  ( -29.17564914869307202, -40.06565635038682416, 12.47384660903968623 ) ) ;
#4870=DIRECTION ( 'NONE',  ( -1.000000000000000000, -0.000000000000000000, -0.000000000000000000 ) ) ;
#4874=VERTEX_POINT ( 'NONE', #5870 ) ;
#4884=CARTESIAN_POINT ( 'NONE',  ( -25.00000000000001776, -45.32948160161801354, 11.45643923738958847 ) ) ;
#4887=CONICAL_SURFACE ( 'NONE', #8122, 1.649999999999998579, 1.029744258676653645 ) ;
#4925=PLANE ( 'NONE',  #6278 ) ;
#4939=CIRCLE ( 'NONE', #5072, 12.49999999999998401 ) ;
#4946=EDGE_CURVE ( 'NONE', #2486, #6859, #1026, .T. ) ;
#4950=CARTESIAN_POINT ( 'NONE',  ( 26.23795701647085821, -41.69067313909253869, 11.92283337402247767 ) ) ;
#4952=LINE ( 'NONE', #7463, #3340 ) ;
#4965=AXIS2_PLACEMENT_3D ( 'NONE', #2342, #4532, #7884 ) ;
#4968=CARTESIAN_POINT ( 'NONE',  ( -29.66610994519569644, -49.99999999999997868, 12.49999999999998401 ) ) ;
#4973=ADVANCED_FACE ( 'NONE', ( #4462 ), #7065, .F. ) ;
#4979=FACE_OUTER_BOUND ( 'NONE', #1677, .T. ) ;
#4986=AXIS2_PLACEMENT_3D ( 'NONE', #1246, #671, #3988 ) ;
#4993=B_SPLINE_CURVE_WITH_KNOTS ( 'NONE', 3,
 ( #1091, #417, #458, #3173, #8541, #7710, #1669, #8502, #2464, #5146, #2509, #4360, #6379, #3871, #6548, #500, #4528, #7214, #1176, #1190 ),
 .UNSPECIFIED., .F., .F.,
 ( 4, 2, 2, 2, 2, 2, 2, 2, 2, 4 ),
 ( 0.000000000000000000, 0.0009878455431463928783, 0.001975691086292775782, 0.002963536629439158469, 0.003951382172585541155, 0.004939227715731924276, 0.005927073258878306529, 0.006420996030451498089, 0.006914918802024691384, 0.007902764345171094454 ),
 .UNSPECIFIED. ) ;
#4995=FACE_OUTER_BOUND ( 'NONE', #3296, .T. ) ;
#4997=DIRECTION ( 'NONE',  ( -0.000000000000000000, -0.000000000000000000, 1.000000000000000000 ) ) ;
#4999=VERTEX_POINT ( 'NONE', #4337 ) ;
#5007=CARTESIAN_POINT ( 'NONE',  ( 31.62327852896863689, -40.25949688271492732, 12.39792973884353344 ) ) ;
#5011=CARTESIAN_POINT ( 'NONE',  ( -28.69222302389759705, -49.83705382567077891, 12.43557624291737795 ) ) ;
#5048=LINE ( 'NONE', #327, #7269 ) ;
#5052=CARTESIAN_POINT ( 'NONE',  ( -27.48298108591646738, -49.33233869400795868, 12.24706002614421507 ) ) ;
#5054=FILL_AREA_STYLE_COLOUR ( '', #3821 ) ;
#5067=ORIENTED_EDGE ( 'NONE', *, *, #5608, .T. ) ;
#5072=AXIS2_PLACEMENT_3D ( 'NONE', #8268, #2319, #1069 ) ;
#5090=CARTESIAN_POINT ( 'NONE',  ( 50.00000000000002842, -44.99999999999997158, 2.099999999999997868 ) ) ;
#5094=CYLINDRICAL_SURFACE ( 'NONE', #1317, 2.099999999999997868 ) ;
#5103=VECTOR ( 'NONE', #1816, 1000.000000000000000 ) ;
#5122=DIRECTION ( 'NONE',  ( -0.000000000000000000, 1.000000000000000000, -0.000000000000000000 ) ) ;
#5136=CARTESIAN_POINT ( 'NONE',  ( -34.99999999999997868, -45.00000000000000000, 11.45643923738958847 ) ) ;
#5138=FILL_AREA_STYLE ('',( #5054 ) ) ;
#5139=ORIENTED_EDGE ( 'NONE', *, *, #2920, .T. ) ;
#5140=PLANE ( 'NONE',  #4414 ) ;
#5146=CARTESIAN_POINT ( 'NONE',  ( -33.76680408720224591, -48.30383393989879437, 11.92131216183668663 ) ) ;
#5150=DIRECTION ( 'NONE',  ( 0.000000000000000000, 0.000000000000000000, 1.000000000000000000 ) ) ;
#5159=DIRECTION ( 'NONE',  ( -0.000000000000000000, 1.000000000000000000, -0.000000000000000000 ) ) ;
#5161=DIRECTION ( 'NONE',  ( -0.000000000000000000, 1.000000000000000000, -0.000000000000000000 ) ) ;
#5166=AXIS2_PLACEMENT_3D ( 'NONE', #7199, #6492, #366 ) ;
#5167=ORIENTED_EDGE ( 'NONE', *, *, #3375, .F. ) ;
#5169=AXIS2_PLACEMENT_3D ( 'NONE', #5543, #125, #739 ) ;
#5173=CARTESIAN_POINT ( 'NONE',  ( 34.32699982994827081, -42.48926715326577863, 11.72748501658993625 ) ) ;
#5187=CARTESIAN_POINT ( 'NONE',  ( -30.00000000000000000, -49.99999999999997158, -12.49999999999997335 ) ) ;
#5188=CARTESIAN_POINT ( 'NONE',  ( -41.99999999999996447, 48.00000000000002842, -22.00000000000000000 ) ) ;
#5190=ORIENTED_EDGE ( 'NONE', *, *, #2254, .F. ) ;
#5199=AXIS2_PLACEMENT_3D ( 'NONE', #7855, #5161, #1820 ) ;
#5201=CARTESIAN_POINT ( 'NONE',  ( -30.00000000000000000, -45.00000000000000000, 30.00000000000000000 ) ) ;
#5211=( GEOMETRIC_REPRESENTATION_CONTEXT ( 3 ) GLOBAL_UNCERTAINTY_ASSIGNED_CONTEXT ( ( #4859 ) ) GLOBAL_UNIT_ASSIGNED_CONTEXT ( ( #372, #7703, #8415 ) ) REPRESENTATION_CONTEXT ( 'NONE', 'WORKASPACE' ) );
#5212=DIRECTION ( 'NONE',  ( 0.000000000000000000, 0.000000000000000000, 1.000000000000000000 ) ) ;
#5216=CARTESIAN_POINT ( 'NONE',  ( 42.00000000000000711, 60.00000000000002842, -23.64999999999992042 ) ) ;
#5222=ORIENTED_EDGE ( 'NONE', *, *, #3659, .F. ) ;
#5224=CARTESIAN_POINT ( 'NONE',  ( -41.99999999999996447, 60.00000000000002842, 22.00000000000000000 ) ) ;
#5233=EDGE_CURVE ( 'NONE', #3140, #58, #101, .T. ) ;
#5258=ORIENTED_EDGE ( 'NONE', *, *, #1937, .F. ) ;
#5265=DIRECTION ( 'NONE',  ( 0.000000000000000000, 0.000000000000000000, 1.000000000000000000 ) ) ;
#5282=CIRCLE ( 'NONE', #1638, 2.099999999999997868 ) ;
#5285=ORIENTED_EDGE ( 'NONE', *, *, #8234, .F. ) ;
#5292=CARTESIAN_POINT ( 'NONE',  ( 34.96649286315892624, -44.33520523457834628, 11.47122145076291666 ) ) ;
#5296=CYLINDRICAL_SURFACE ( 'NONE', #7515, 12.49999999999997691 ) ;
#5305=AXIS2_PLACEMENT_3D ( 'NONE', #3189, #4997, #1645 ) ;
#5310=CARTESIAN_POINT ( 'NONE',  ( 30.00000000000001421, -44.99999999999995737, 30.00000000000000000 ) ) ;
#5315=ORIENTED_EDGE ( 'NONE', *, *, #1884, .F. ) ;
#5325=EDGE_CURVE ( 'NONE', #8403, #4829, #556, .T. ) ;
#5336=DIRECTION ( 'NONE',  ( 0.000000000000000000, 0.000000000000000000, 1.000000000000000000 ) ) ;
#5342=ORIENTED_EDGE ( 'NONE', *, *, #8374, .F. ) ;
#5348=ORIENTED_EDGE ( 'NONE', *, *, #5325, .F. ) ;
#5349=ORIENTED_EDGE ( 'NONE', *, *, #5570, .T. ) ;
#5357=( GEOMETRIC_REPRESENTATION_CONTEXT ( 3 ) GLOBAL_UNCERTAINTY_ASSIGNED_CONTEXT ( ( #4064 ) ) GLOBAL_UNIT_ASSIGNED_CONTEXT ( ( #7121, #4518, #7872 ) ) REPRESENTATION_CONTEXT ( 'NONE', 'WORKASPACE' ) );
#5361=ORIENTED_EDGE ( 'NONE', *, *, #3375, .T. ) ;
#5368=EDGE_CURVE ( 'NONE', #2514, #1305, #7845, .T. ) ;
#5373=EDGE_LOOP ( 'NONE', ( #2067, #279, #3869 ) ) ;
#5374=DIRECTION ( 'NONE',  ( 1.000000000000000000, 0.000000000000000000, 0.000000000000000000 ) ) ;
#5378=AXIS2_PLACEMENT_3D ( 'NONE', #5310, #5265, #7299 ) ;
#5392=ORIENTED_EDGE ( 'NONE', *, *, #1539, .F. ) ;
#5395=CARTESIAN_POINT ( 'NONE',  ( -49.99999999999997158, 60.00000000000002842, 30.00000000000000000 ) ) ;
#5403=ORIENTED_EDGE ( 'NONE', *, *, #3019, .F. ) ;
#5414=CIRCLE ( 'NONE', #5985, 1.649999999999998579 ) ;
#5416=CARTESIAN_POINT ( 'NONE',  ( 28.37383639613264208, -49.73950299483291104, 12.39754634550704182 ) ) ;
#5417=DIRECTION ( 'NONE',  ( -0.000000000000000000, 1.000000000000000000, -0.000000000000000000 ) ) ;
#5425=CARTESIAN_POINT ( 'NONE',  ( -25.25873964592378229, -43.37909215248190264, 11.56670877700491040 ) ) ;
#5429=CARTESIAN_POINT ( 'NONE',  ( 50.00000000000002842, -59.99999999999997158, -30.00000000000000000 ) ) ;
#5437=ORIENTED_EDGE ( 'NONE', *, *, #2472, .T. ) ;
#5441=DIRECTION ( 'NONE',  ( -0.000000000000000000, -1.000000000000000000, -0.000000000000000000 ) ) ;
#5442=CARTESIAN_POINT ( 'NONE',  ( -25.00000000000002487, -45.00000000000000000, 11.45643923738959025 ) ) ;
#5478=EDGE_CURVE ( 'NONE', #2602, #8290, #988, .T. ) ;
#5481=CONICAL_SURFACE ( 'NONE', #7461, 12.49999999999996980, 1.029744258676651869 ) ;
#5482=VERTEX_POINT ( 'NONE', #3984 ) ;
#5490=CARTESIAN_POINT ( 'NONE',  ( 0.000000000000000000, 0.000000000000000000, 30.00000000000000000 ) ) ;
#5506=CARTESIAN_POINT ( 'NONE',  ( -41.99999999999996447, 60.00000000000002842, -20.35000000000000142 ) ) ;
#5512=FACE_OUTER_BOUND ( 'NONE', #868, .T. ) ;
#5516=CARTESIAN_POINT ( 'NONE',  ( -25.44732502511945782, -42.92638634940919928, 11.64163759925511599 ) ) ;
#5522=AXIS2_PLACEMENT_3D ( 'NONE', #2467, #7217, #8425 ) ;
#5524=DIRECTION ( 'NONE',  ( 0.000000000000000000, -0.000000000000000000, 1.000000000000000000 ) ) ;
#5526=AXIS2_PLACEMENT_3D ( 'NONE', #2682, #4615, #8053 ) ;
#5532=AXIS2_PLACEMENT_3D ( 'NONE', #7207, #4440, #5844 ) ;
#5533=CARTESIAN_POINT ( 'NONE',  ( 43.73819270004214843, -44.99999999999997158, 0.000000000000000000 ) ) ;
#5541=ORIENTED_EDGE ( 'NONE', *, *, #6794, .F. ) ;
#5543=CARTESIAN_POINT ( 'NONE',  ( -30.00000000000000000, 60.00000000000002842, 0.000000000000000000 ) ) ;
#5547=CARTESIAN_POINT ( 'NONE',  ( 50.00000000000002842, -59.99999999999997158, 30.00000000000000000 ) ) ;
#5558=CARTESIAN_POINT ( 'NONE',  ( -28.37672147103137732, -40.25949688271495575, 12.39792973884354232 ) ) ;
#5559=DIRECTION ( 'NONE',  ( -0.000000000000000000, 1.000000000000000000, -0.000000000000000000 ) ) ;
#5564=PLANE ( 'NONE',  #4178 ) ;
#5570=EDGE_CURVE ( 'NONE', #8403, #8204, #7272, .T. ) ;
#5576=CARTESIAN_POINT ( 'NONE',  ( -25.51052057033350096, -47.22506321083132974, 11.66673928690326179 ) ) ;
#5577=FACE_BOUND ( 'NONE', #8468, .T. ) ;
#5579=AXIS2_PLACEMENT_3D ( 'NONE', #3637, #3551, #5824 ) ;
#5580=EDGE_CURVE ( 'NONE', #2059, #5916, #947, .T. ) ;
#5588=EDGE_CURVE ( 'NONE', #8058, #1053, #3068, .T. ) ;
#5593=AXIS2_PLACEMENT_3D ( 'NONE', #3573, #1622, #784 ) ;
#5602=DIRECTION ( 'NONE',  ( -0.000000000000000000, 1.000000000000000000, -0.000000000000000000 ) ) ;
#5604=CARTESIAN_POINT ( 'NONE',  ( -26.23123798130810158, -41.69806059905386064, 11.92074493419280756 ) ) ;
#5608=EDGE_CURVE ( 'NONE', #4084, #4999, #7707, .T. ) ;
#5614=VERTEX_POINT ( 'NONE', #7377 ) ;
#5620=CARTESIAN_POINT ( 'NONE',  ( -34.48648245112668320, -42.76835092305881858, 11.66791272636412913 ) ) ;
#5624=B_SPLINE_CURVE_WITH_KNOTS ( 'NONE', 3,
 ( #6068, #3306, #8584, #6727, #7302, #6024, #4002, #1303, #548, #7393, #4709, #686, #3874, #3257, #5980, #2551, #7969, #8673 ),
 .UNSPECIFIED., .F., .F.,
 ( 4, 2, 2, 2, 2, 2, 2, 2, 4 ),
 ( 0.02369462427231871365, 0.02468136329545927640, 0.02566810231859983568, 0.02665484134174039843, 0.02764158036488095771, 0.02862831938802152046, 0.02961505841116208321, 0.03060179743430264249, 0.03158853645744319483 ),
 .UNSPECIFIED. ) ;
#5644=DIRECTION ( 'NONE',  ( 0.000000000000000000, 0.000000000000000000, 1.000000000000000000 ) ) ;
#5647=EDGE_CURVE ( 'NONE', #4635, #1100, #6048, .T. ) ;
#5660=CONICAL_SURFACE ( 'NONE', #6503, 2.099999999999997868, 1.029744258676652313 ) ;
#5673=CIRCLE ( 'NONE', #7082, 4.999999999999969802 ) ;
#5674=ORIENTED_EDGE ( 'NONE', *, *, #6794, .T. ) ;
#5685=EDGE_CURVE ( 'NONE', #1617, #3140, #6575, .T. ) ;
#5699=VERTEX_POINT ( 'NONE', #3935 ) ;
#5700=ORIENTED_EDGE ( 'NONE', *, *, #2998, .T. ) ;
#5709=PRODUCT_DEFINITION_SHAPE ( 'NONE', 'NONE',  #2881 ) ;
#5734=CYLINDRICAL_SURFACE ( 'NONE', #4805, 2.099999999999997868 ) ;
#5740=LINE ( 'NONE', #4624, #481 ) ;
#5743=ADVANCED_FACE ( 'NONE', ( #1951 ), #1372, .F. ) ;
#5744=FACE_OUTER_BOUND ( 'NONE', #2348, .T. ) ;
#5751=CARTESIAN_POINT ( 'NONE',  ( 30.32909313480922009, -40.00809359540121335, 12.49675575313100850 ) ) ;
#5754=FACE_OUTER_BOUND ( 'NONE', #4164, .T. ) ;
#5761=EDGE_CURVE ( 'NONE', #8500, #7164, #8035, .T. ) ;
#5762=EDGE_LOOP ( 'NONE', ( #1526, #3218, #6301, #2344 ) ) ;
#5772=CIRCLE ( 'NONE', #8319, 2.099999999999997868 ) ;
#5777=VECTOR ( 'NONE', #2801, 1000.000000000000000 ) ;
#5778=CARTESIAN_POINT ( 'NONE',  ( 34.99999999999998579, -44.99999999999995737, 11.45643923738957071 ) ) ;
#5782=CARTESIAN_POINT ( 'NONE',  ( -41.99999999999996447, 60.00000000000002842, 22.00000000000000000 ) ) ;
#5784=DIRECTION ( 'NONE',  ( 0.000000000000000000, 0.5150380749100563760, 0.8571673007021110013 ) ) ;
#5796=DIRECTION ( 'NONE',  ( -0.000000000000000000, -0.000000000000000000, 1.000000000000000000 ) ) ;
#5801=DIRECTION ( 'NONE',  ( 0.000000000000000000, 0.000000000000000000, 1.000000000000000000 ) ) ;
#5819=VERTEX_POINT ( 'NONE', #1324 ) ;
#5824=DIRECTION ( 'NONE',  ( 0.000000000000000000, 0.000000000000000000, 1.000000000000000000 ) ) ;
#5825=DIRECTION ( 'NONE',  ( 0.000000000000000000, 0.000000000000000000, 1.000000000000000000 ) ) ;
#5831=EDGE_LOOP ( 'NONE', ( #8286, #7004, #7134, #1648 ) ) ;
#5836=CARTESIAN_POINT ( 'NONE',  ( 33.97336238306395728, -41.94765302695299169, 11.85321826485148655 ) ) ;
#5843=ORIENTED_EDGE ( 'NONE', *, *, #4849, .T. ) ;
#5844=DIRECTION ( 'NONE',  ( 0.000000000000000000, 0.000000000000000000, 1.000000000000000000 ) ) ;
#5847=ORIENTED_EDGE ( 'NONE', *, *, #5647, .T. ) ;
#5858=AXIS2_PLACEMENT_3D ( 'NONE', #70, #3523, #7479 ) ;
#5859=CONICAL_SURFACE ( 'NONE', #7544, 2.099999999999997868, 1.029744258676652313 ) ;
#5860=EDGE_CURVE ( 'NONE', #4874, #8058, #1995, .T. ) ;
#5861=ORIENTED_EDGE ( 'NONE', *, *, #2103, .T. ) ;
#5866=FACE_OUTER_BOUND ( 'NONE', #6596, .T. ) ;
#5870=CARTESIAN_POINT ( 'NONE',  ( 42.00000000000000711, 48.00000000000002842, 20.34999999999992326 ) ) ;
#5872=AXIS2_PLACEMENT_3D ( 'NONE', #3199, #7998, #668 ) ;
#5894=ORIENTED_EDGE ( 'NONE', *, *, #3769, .T. ) ;
#5897=CARTESIAN_POINT ( 'NONE',  ( -41.99999999999996447, 60.00000000000002842, -23.64999999999999858 ) ) ;
#5916=VERTEX_POINT ( 'NONE', #885 ) ;
#5933=EDGE_LOOP ( 'NONE', ( #1920, #2235, #7802 ) ) ;
#5957=ADVANCED_FACE ( 'NONE', ( #5512 ), #2295, .F. ) ;
#5962=CIRCLE ( 'NONE', #6662, 2.099999999999997868 ) ;
#5967=LINE ( 'NONE', #7870, #8375 ) ;
#5969=EDGE_LOOP ( 'NONE', ( #8247, #8459, #5067 ) ) ;
#5972=ADVANCED_FACE ( 'NONE', ( #2136 ), #8221, .T. ) ;
#5980=CARTESIAN_POINT ( 'NONE',  ( 31.30777697610241006, -49.83705382567072917, 12.43557624291735841 ) ) ;
#5982=VERTEX_POINT ( 'NONE', #6966 ) ;
#5985=AXIS2_PLACEMENT_3D ( 'NONE', #4690, #2139, #6882 ) ;
#5986=ORIENTED_EDGE ( 'NONE', *, *, #2951, .T. ) ;
#5995=CARTESIAN_POINT ( 'NONE',  ( 29.33771720961957641, -49.96682304584948753, 12.48662461771946397 ) ) ;
#5996=VECTOR ( 'NONE', #6804, 1000.000000000000000 ) ;
#6006=DIRECTION ( 'NONE',  ( -0.000000000000000000, 1.000000000000000000, -0.000000000000000000 ) ) ;
#6009=CYLINDRICAL_SURFACE ( 'NONE', #4556, 12.49999999999998046 ) ;
#6022=DIRECTION ( 'NONE',  ( -1.000000000000000000, -0.000000000000000000, -0.000000000000000000 ) ) ;
#6024=CARTESIAN_POINT ( 'NONE',  ( 34.48947942966652391, -47.22506321083128711, 11.66673928690324225 ) ) ;
#6048=LINE ( 'NONE', #7950, #8550 ) ;
#6054=CONICAL_SURFACE ( 'NONE', #7318, 1.649999999999998579, 1.029744258676653645 ) ;
#6055=VERTEX_POINT ( 'NONE', #4156 ) ;
#6060=EDGE_CURVE ( 'NONE', #4635, #912, #6834, .T. ) ;
#6065=SURFACE_STYLE_FILL_AREA ( #3999 ) ;
#6068=CARTESIAN_POINT ( 'NONE',  ( 34.99999999999998579, -44.99999999999995737, 11.45643923738957071 ) ) ;
#6070=VERTEX_POINT ( 'NONE', #7104 ) ;
#6075=EDGE_LOOP ( 'NONE', ( #6817, #3911, #8534, #1278 ) ) ;
#6083=EDGE_CURVE ( 'NONE', #5819, #3280, #1016, .T. ) ;
#6087=CARTESIAN_POINT ( 'NONE',  ( 25.26672068143954064, -46.61962928414787655, 11.56930355017052037 ) ) ;
#6107=ORIENTED_EDGE ( 'NONE', *, *, #4946, .F. ) ;
#6113=CARTESIAN_POINT ( 'NONE',  ( 42.00000000000000711, 48.00000000000002842, -21.99999999999992184 ) ) ;
#6136=CARTESIAN_POINT ( 'NONE',  ( 42.00000000000000711, 60.00000000000002842, 20.34999999999992326 ) ) ;
#6142=AXIS2_PLACEMENT_3D ( 'NONE', #6883, #4870, #7632 ) ;
#6145=CARTESIAN_POINT ( 'NONE',  ( 45.00000000000003553, -44.99999999999997158, 2.099999999999997868 ) ) ;
#6180=B_SPLINE_CURVE_WITH_KNOTS ( 'NONE', 3,
 ( #6813, #4840, #7560, #2284, #7476, #5620, #907, #6855, #4216, #7519, #3562, #4261, #8152, #1479, #1565, #6246, #3477, #6986, #4301, #3602 ),
 .UNSPECIFIED., .F., .F.,
 ( 4, 2, 2, 2, 2, 2, 2, 2, 2, 4 ),
 ( 0.007902764345171094454, 0.008889850383257352426, 0.009876936421343610398, 0.01086402245942986837, 0.01185110849751612634, 0.01283819453560238258, 0.01333173755464549942, 0.01382528057368861280, 0.01481236661177484301, 0.01579945264986107323 ),
 .UNSPECIFIED. ) ;
#6183=CARTESIAN_POINT ( 'NONE',  ( -25.75674496862487572, -42.35030295949449197, 11.75814120956406050 ) ) ;
#6184=CARTESIAN_POINT ( 'NONE',  ( 45.00000000000003553, -44.99999999999997158, -2.099999999999997868 ) ) ;
#6188=ORIENTED_EDGE ( 'NONE', *, *, #1546, .T. ) ;
#6189=DIRECTION ( 'NONE',  ( 0.000000000000000000, 1.000000000000000000, 0.000000000000000000 ) ) ;
#6190=ORIENTED_EDGE ( 'NONE', *, *, #6608, .T. ) ;
#6201=FACE_OUTER_BOUND ( 'NONE', #625, .T. ) ;
#6222=CARTESIAN_POINT ( 'NONE',  ( -41.99999999999996447, 48.00000000000002842, -22.00000000000000000 ) ) ;
#6226=CARTESIAN_POINT ( 'NONE',  ( 28.68975157273829169, -40.16330870357082716, 12.43543189630222656 ) ) ;
#6229=ADVANCED_FACE ( 'NONE', ( #5866 ), #5660, .F. ) ;
#6235=VERTEX_POINT ( 'NONE', #2521 ) ;
#6246=CARTESIAN_POINT ( 'NONE',  ( -31.62280801364509486, -40.25948930238543966, 12.39794155511765794 ) ) ;
#6269=CARTESIAN_POINT ( 'NONE',  ( -29.83554193206648009, -40.00000000000002132, 12.49999999999998046 ) ) ;
#6276=ORIENTED_EDGE ( 'NONE', *, *, #1937, .T. ) ;
#6278=AXIS2_PLACEMENT_3D ( 'NONE', #247, #7563, #2114 ) ;
#6286=DIRECTION ( 'NONE',  ( -0.000000000000000000, 1.000000000000000000, -0.000000000000000000 ) ) ;
#6288=VERTEX_POINT ( 'NONE', #5547 ) ;
#6301=ORIENTED_EDGE ( 'NONE', *, *, #5368, .T. ) ;
#6332=APPLICATION_CONTEXT ( 'automotive_design' ) ;
#6337=LINE ( 'NONE', #2253, #4018 ) ;
#6348=FACE_OUTER_BOUND ( 'NONE', #4428, .T. ) ;
#6354=CARTESIAN_POINT ( 'NONE',  ( 30.00000000000000000, -49.99999999999997158, -1.102182119232617753E-14 ) ) ;
#6379=CARTESIAN_POINT ( 'NONE',  ( -34.49011023859264924, -47.22366675470355091, 11.66649199791333125 ) ) ;
#6385=VERTEX_POINT ( 'NONE', #2212 ) ;
#6398=EDGE_CURVE ( 'NONE', #8668, #4874, #2006, .T. ) ;
#6413=DIRECTION ( 'NONE',  ( -0.000000000000000000, 1.000000000000000000, -0.000000000000000000 ) ) ;
#6416=VERTEX_POINT ( 'NONE', #1625 ) ;
#6425=LINE ( 'NONE', #5187, #2152 ) ;
#6429=ORIENTED_EDGE ( 'NONE', *, *, #4029, .T. ) ;
#6439=DIRECTION ( 'NONE',  ( 0.000000000000000000, 0.000000000000000000, 1.000000000000000000 ) ) ;
#6446=EDGE_LOOP ( 'NONE', ( #4772, #7708, #6190 ) ) ;
#6453=FACE_OUTER_BOUND ( 'NONE', #3571, .T. ) ;
#6454=DIRECTION ( 'NONE',  ( -1.000000000000000000, -0.000000000000000000, -0.000000000000000000 ) ) ;
#6457=ORIENTED_EDGE ( 'NONE', *, *, #1924, .T. ) ;
#6458=DIRECTION ( 'NONE',  ( -0.000000000000000000, 1.000000000000000000, -0.000000000000000000 ) ) ;
#6461=ORIENTED_EDGE ( 'NONE', *, *, #5588, .F. ) ;
#6476=DIRECTION ( 'NONE',  ( 0.000000000000000000, 0.000000000000000000, 1.000000000000000000 ) ) ;
#6482=MECHANICAL_DESIGN_GEOMETRIC_PRESENTATION_REPRESENTATION('',(#302),#5357);
#6486=ORIENTED_EDGE ( 'NONE', *, *, #6490, .T. ) ;
#6490=EDGE_CURVE ( 'NONE', #6385, #6859, #32, .T. ) ;
#6492=DIRECTION ( 'NONE',  ( -0.000000000000000000, 1.000000000000000000, -0.000000000000000000 ) ) ;
#6503=AXIS2_PLACEMENT_3D ( 'NONE', #8434, #2397, #6439 ) ;
#6508=CARTESIAN_POINT ( 'NONE',  ( 42.00000000000000711, 47.00857997860455129, 21.99999999999992184 ) ) ;
#6510=EDGE_LOOP ( 'NONE', ( #5392, #983 ) ) ;
#6513=EDGE_CURVE ( 'NONE', #8204, #5819, #7713, .T. ) ;
#6520=ADVANCED_FACE ( 'NONE', ( #7173 ), #3424, .F. ) ;
#6521=VECTOR ( 'NONE', #6815, 1000.000000000000000 ) ;
#6529=VERTEX_POINT ( 'NONE', #1134 ) ;
#6541=DIRECTION ( 'NONE',  ( 0.000000000000000000, 0.000000000000000000, -1.000000000000000000 ) ) ;
#6547=AXIS2_PLACEMENT_3D ( 'NONE', #6549, #1716, #3130 ) ;
#6548=CARTESIAN_POINT ( 'NONE',  ( -34.73327931856048423, -46.61962928414794760, 11.56930355017053280 ) ) ;
#6549=CARTESIAN_POINT ( 'NONE',  ( -41.99999999999996447, 60.00000000000002842, 22.00000000000000000 ) ) ;
#6550=CARTESIAN_POINT ( 'NONE',  ( 50.00000000000002842, 60.00000000000002842, 30.00000000000000000 ) ) ;
#6557=VERTEX_POINT ( 'NONE', #6508 ) ;
#6558=ADVANCED_FACE ( 'NONE', ( #8505, #7093 ), #4363, .F. ) ;
#6568=LINE ( 'NONE', #1236, #880 ) ;
#6574=DIRECTION ( 'NONE',  ( 0.000000000000000000, 0.000000000000000000, 1.000000000000000000 ) ) ;
#6575=LINE ( 'NONE', #2046, #801 ) ;
#6591=DIRECTION ( 'NONE',  ( 0.000000000000000000, 0.000000000000000000, 1.000000000000000000 ) ) ;
#6596=EDGE_LOOP ( 'NONE', ( #7704, #5847, #6429 ) ) ;
#6597=DIRECTION ( 'NONE',  ( -0.000000000000000000, 1.000000000000000000, -0.000000000000000000 ) ) ;
#6608=EDGE_CURVE ( 'NONE', #5916, #2059, #8349, .T. ) ;
#6616=LINE ( 'NONE', #8656, #2200 ) ;
#6620=DIRECTION ( 'NONE',  ( -0.000000000000000000, 1.000000000000000000, -0.000000000000000000 ) ) ;
#6623=ORIENTED_EDGE ( 'NONE', *, *, #3777, .F. ) ;
#6628=ORIENTED_EDGE ( 'NONE', *, *, #7092, .T. ) ;
#6629=EDGE_LOOP ( 'NONE', ( #523, #4744 ) ) ;
#6632=DIRECTION ( 'NONE',  ( -0.000000000000000000, 1.000000000000000000, -0.000000000000000000 ) ) ;
#6637=ORIENTED_EDGE ( 'NONE', *, *, #2771, .F. ) ;
#6650=EDGE_CURVE ( 'NONE', #1784, #2059, #2512, .T. ) ;
#6657=ORIENTED_EDGE ( 'NONE', *, *, #995, .T. ) ;
#6662=AXIS2_PLACEMENT_3D ( 'NONE', #4436, #8490, #3815 ) ;
#6672=LINE ( 'NONE', #626, #5996 ) ;
#6679=DIRECTION ( 'NONE',  ( -0.000000000000000000, 1.000000000000000000, -0.000000000000000000 ) ) ;
#6680=CARTESIAN_POINT ( 'NONE',  ( -45.00000000000003553, -44.99999999999997158, 2.099999999999997868 ) ) ;
#6688=ORIENTED_EDGE ( 'NONE', *, *, #7805, .T. ) ;
#6698=DIRECTION ( 'NONE',  ( 1.000000000000000000, 0.000000000000000000, 0.000000000000000000 ) ) ;
#6711=FACE_OUTER_BOUND ( 'NONE', #139, .T. ) ;
#6716=CARTESIAN_POINT ( 'NONE',  ( 30.00000000000000000, 60.00000000000002842, 12.49999999999997335 ) ) ;
#6727=CARTESIAN_POINT ( 'NONE',  ( 34.83728160242328187, -46.30802241892373416, 11.52630626327733410 ) ) ;
#6748=CIRCLE ( 'NONE', #3668, 1.649999999999998579 ) ;
#6760=CIRCLE ( 'NONE', #857, 12.49999999999996980 ) ;
#6768=ORIENTED_EDGE ( 'NONE', *, *, #8065, .T. ) ;
#6786=CARTESIAN_POINT ( 'NONE',  ( 25.50988976140734366, -47.22366675470350117, 11.66649199791332592 ) ) ;
#6790=ORIENTED_EDGE ( 'NONE', *, *, #495, .F. ) ;
#6794=EDGE_CURVE ( 'NONE', #8290, #8403, #5624, .T. ) ;
#6801=CIRCLE ( 'NONE', #5532, 1.649999999999998579 ) ;
#6804=DIRECTION ( 'NONE',  ( -1.000000000000000000, -0.000000000000000000, -0.000000000000000000 ) ) ;
#6809=SHAPE_REPRESENTATION ( 'Body', ( #2554 ), #5211 ) ;
#6813=CARTESIAN_POINT ( 'NONE',  ( -34.99999999999997868, -45.00000000000000000, 11.45643923738958847 ) ) ;
#6815=DIRECTION ( 'NONE',  ( -0.000000000000000000, -0.000000000000000000, 1.000000000000000000 ) ) ;
#6816=DIRECTION ( 'NONE',  ( 0.000000000000000000, 0.000000000000000000, 1.000000000000000000 ) ) ;
#6817=ORIENTED_EDGE ( 'NONE', *, *, #4327, .T. ) ;
#6834=LINE ( 'NONE', #8392, #5103 ) ;
#6837=CARTESIAN_POINT ( 'NONE',  ( 25.03353697015359458, -44.33501760501477662, 11.47123432380332808 ) ) ;
#6845=VERTEX_POINT ( 'NONE', #3392 ) ;
#6847=ORIENTED_EDGE ( 'NONE', *, *, #3921, .F. ) ;
#6852=ORIENTED_EDGE ( 'NONE', *, *, #7534, .F. ) ;
#6855=CARTESIAN_POINT ( 'NONE',  ( -33.97112193926510315, -41.94466314146776398, 11.85397847079114975 ) ) ;
#6859=VERTEX_POINT ( 'NONE', #1347 ) ;
#6879=CARTESIAN_POINT ( 'NONE',  ( -30.00000000000000000, -45.00000000000000000, 30.00000000000000000 ) ) ;
#6882=DIRECTION ( 'NONE',  ( 0.000000000000000000, 0.000000000000000000, 1.000000000000000000 ) ) ;
#6883=CARTESIAN_POINT ( 'NONE',  ( -50.00000000000002842, -44.99999999999997158, 0.000000000000000000 ) ) ;
#6887=ORIENTED_EDGE ( 'NONE', *, *, #5860, .T. ) ;
#6888=FACE_OUTER_BOUND ( 'NONE', #3368, .T. ) ;
#6889=ORIENTED_EDGE ( 'NONE', *, *, #5761, .F. ) ;
#6902=DIRECTION ( 'NONE',  ( 0.000000000000000000, 0.000000000000000000, 1.000000000000000000 ) ) ;
#6903=ORIENTED_EDGE ( 'NONE', *, *, #495, .T. ) ;
#6906=VECTOR ( 'NONE', #268, 1000.000000000000000 ) ;
#6926=CARTESIAN_POINT ( 'NONE',  ( -26.94291110594769734, -41.03022111473443090, 12.12354317000653836 ) ) ;
#6927=DIRECTION ( 'NONE',  ( 0.5150380749100560429, 0.000000000000000000, -0.8571673007021112234 ) ) ;
#6934=LINE ( 'NONE', #1602, #1076 ) ;
#6935=ORIENTED_EDGE ( 'NONE', *, *, #3126, .F. ) ;
#6966=CARTESIAN_POINT ( 'NONE',  ( 29.99999999999997158, -57.51075773784449296, -1.102182119232617753E-14 ) ) ;
#6968=VECTOR ( 'NONE', #962, 1000.000000000000000 ) ;
#6969=CARTESIAN_POINT ( 'NONE',  ( -29.67090686519078346, -40.00809359540125598, 12.49675575313102271 ) ) ;
#6979=AXIS2_PLACEMENT_3D ( 'NONE', #2777, #6286, #6902 ) ;
#6982=AXIS2_PLACEMENT_3D ( 'NONE', #8226, #2799, #54 ) ;
#6986=CARTESIAN_POINT ( 'NONE',  ( -30.65892580703207670, -40.03249052150655274, 12.48689449661284279 ) ) ;
#6996=CARTESIAN_POINT ( 'NONE',  ( 50.00000000000002842, -44.99999999999997158, 2.099999999999997868 ) ) ;
#7004=ORIENTED_EDGE ( 'NONE', *, *, #1924, .F. ) ;
#7022=ORIENTED_EDGE ( 'NONE', *, *, #3749, .T. ) ;
#7033=VECTOR ( 'NONE', #2585, 1000.000000000000000 ) ;
#7040=AXIS2_PLACEMENT_3D ( 'NONE', #4392, #1876, #7160 ) ;
#7056=B_SPLINE_CURVE_WITH_KNOTS ( 'NONE', 3,
 ( #2270, #1420, #6837, #845, #2227, #228, #3589, #1507, #4950, #53, #4201, #3545, #1465, #4286, #7588, #2842, #6226, #187, #805, #2798 ),
 .UNSPECIFIED., .F., .F.,
 ( 4, 2, 2, 2, 2, 2, 2, 2, 2, 4 ),
 ( 0.007902764345171071902, 0.008889850383257314262, 0.009876936421343554887, 0.01086402245942979725, 0.01185110849751603787, 0.01283819453560228023, 0.01333173755464540575, 0.01382528057368853300, 0.01481236661177478577, 0.01579945264986103853 ),
 .UNSPECIFIED. ) ;
#7065=CYLINDRICAL_SURFACE ( 'NONE', #5305, 4.999999999999973355 ) ;
#7068=VECTOR ( 'NONE', #3088, 1000.000000000000000 ) ;
#7069=ORIENTED_EDGE ( 'NONE', *, *, #8065, .F. ) ;
#7070=EDGE_CURVE ( 'NONE', #8290, #207, #7562, .T. ) ;
#7077=CARTESIAN_POINT ( 'NONE',  ( 30.16445806793351636, -39.99999999999998579, 12.49999999999996625 ) ) ;
#7081=DIRECTION ( 'NONE',  ( 0.000000000000000000, 0.000000000000000000, 1.000000000000000000 ) ) ;
#7082=AXIS2_PLACEMENT_3D ( 'NONE', #8194, #4215, #2283 ) ;
#7084=CARTESIAN_POINT ( 'NONE',  ( 42.00000000000000711, 48.00000000000002842, 23.64999999999992042 ) ) ;
#7092=EDGE_CURVE ( 'NONE', #2769, #6055, #8197, .T. ) ;
#7093=FACE_OUTER_BOUND ( 'NONE', #6075, .T. ) ;
#7104=CARTESIAN_POINT ( 'NONE',  ( 50.00000000000002842, -59.99999999999997158, -30.00000000000000000 ) ) ;
#7108=DIRECTION ( 'NONE',  ( 0.000000000000000000, 0.000000000000000000, 1.000000000000000000 ) ) ;
#7121=( LENGTH_UNIT ( ) NAMED_UNIT ( * ) SI_UNIT ( .MILLI., .METRE. ) );
#7122=ORIENTED_EDGE ( 'NONE', *, *, #8340, .F. ) ;
#7126=ORIENTED_EDGE ( 'NONE', *, *, #5588, .T. ) ;
#7134=ORIENTED_EDGE ( 'NONE', *, *, #1692, .T. ) ;
#7160=DIRECTION ( 'NONE',  ( 0.000000000000000000, 0.000000000000000000, 1.000000000000000000 ) ) ;
#7161=FACE_OUTER_BOUND ( 'NONE', #8606, .T. ) ;
#7164=VERTEX_POINT ( 'NONE', #8241 ) ;
#7168=EDGE_LOOP ( 'NONE', ( #346, #5403 ) ) ;
#7172=LINE ( 'NONE', #6550, #3696 ) ;
#7173=FACE_OUTER_BOUND ( 'NONE', #6446, .T. ) ;
#7175=EDGE_CURVE ( 'NONE', #1617, #6859, #2477, .T. ) ;
#7180=AXIS2_PLACEMENT_3D ( 'NONE', #1067, #1643, #356 ) ;
#7189=CARTESIAN_POINT ( 'NONE',  ( 42.00000000000000711, 48.00000000000002842, -21.99999999999992184 ) ) ;
#7199=CARTESIAN_POINT ( 'NONE',  ( -41.99999999999996447, 60.00000000000002842, -22.00000000000000000 ) ) ;
#7202=CARTESIAN_POINT ( 'NONE',  ( -34.99999999999997868, -45.00000000000000000, -30.00100000000000122 ) ) ;
#7203=DIRECTION ( 'NONE',  ( 1.000000000000000000, -0.000000000000000000, -0.000000000000000000 ) ) ;
#7207=CARTESIAN_POINT ( 'NONE',  ( -41.99999999999996447, 60.00000000000002842, -22.00000000000000000 ) ) ;
#7210=EDGE_CURVE ( 'NONE', #4999, #4084, #5962, .T. ) ;
#7214=CARTESIAN_POINT ( 'NONE',  ( -34.96759668750374317, -45.65721116879225860, 11.47074269425085724 ) ) ;
#7217=DIRECTION ( 'NONE',  ( -0.000000000000000000, 1.000000000000000000, -0.000000000000000000 ) ) ;
#7221=CIRCLE ( 'NONE', #8360, 12.49999999999998757 ) ;
#7222=EDGE_LOOP ( 'NONE', ( #2673, #491, #373 ) ) ;
#7235=ORIENTED_EDGE ( 'NONE', *, *, #3131, .F. ) ;
#7241=DIRECTION ( 'NONE',  ( -0.000000000000000000, 1.000000000000000000, -0.000000000000000000 ) ) ;
#7244=DIRECTION ( 'NONE',  ( -0.000000000000000000, 1.000000000000000000, -0.000000000000000000 ) ) ;
#7245=LINE ( 'NONE', #5216, #1598 ) ;
#7247=ORIENTED_EDGE ( 'NONE', *, *, #7805, .F. ) ;
#7252=EDGE_CURVE ( 'NONE', #6055, #6288, #2416, .T. ) ;
#7253=EDGE_LOOP ( 'NONE', ( #253, #1667, #5861, #2650, #3248 ) ) ;
#7255=AXIS2_PLACEMENT_3D ( 'NONE', #1242, #8088, #6574 ) ;
#7262=ADVANCED_FACE ( 'NONE', ( #290 ), #3732, .F. ) ;
#7269=VECTOR ( 'NONE', #1700, 1000.000000000000000 ) ;
#7272=CIRCLE ( 'NONE', #7556, 12.49999999999996980 ) ;
#7276=CARTESIAN_POINT ( 'NONE',  ( 30.00000000000001421, -44.99999999999995737, -30.00100000000000122 ) ) ;
#7279=VERTEX_POINT ( 'NONE', #5136 ) ;
#7280=CARTESIAN_POINT ( 'NONE',  ( -30.00000000000000000, -45.00000000000000000, -30.00100000000000122 ) ) ;
#7289=DIRECTION ( 'NONE',  ( 0.000000000000000000, 0.000000000000000000, 1.000000000000000000 ) ) ;
#7297=ORIENTED_EDGE ( 'NONE', *, *, #1884, .T. ) ;
#7299=DIRECTION ( 'NONE',  ( -1.000000000000000000, 0.000000000000000000, 0.000000000000000000 ) ) ;
#7300=CARTESIAN_POINT ( 'NONE',  ( -41.99999999999996447, 48.00000000000002842, 22.00000000000000000 ) ) ;
#7302=CARTESIAN_POINT ( 'NONE',  ( 34.74044648917334399, -46.62311395930098712, 11.56703930231303978 ) ) ;
#7307=ORIENTED_EDGE ( 'NONE', *, *, #3215, .F. ) ;
#7312=CARTESIAN_POINT ( 'NONE',  ( 42.00000000000000711, 47.00857997860455129, -21.99999999999992184 ) ) ;
#7313=ADVANCED_FACE ( 'NONE', ( #7161 ), #46, .F. ) ;
#7315=CONICAL_SURFACE ( 'NONE', #7180, 1.649999999999998579, 1.029744258676653645 ) ;
#7318=AXIS2_PLACEMENT_3D ( 'NONE', #1379, #7244, #1916 ) ;
#7329=CARTESIAN_POINT ( 'NONE',  ( 34.74126035407623192, -43.37909215248186712, 11.56670877700489264 ) ) ;
#7333=CYLINDRICAL_SURFACE ( 'NONE', #4986, 1.649999999999998579 ) ;
#7345=CARTESIAN_POINT ( 'NONE',  ( -49.99999999999997158, 60.00000000000002842, 30.00000000000000000 ) ) ;
#7354=ADVANCED_FACE ( 'NONE', ( #5754 ), #5094, .F. ) ;
#7369=ORIENTED_EDGE ( 'NONE', *, *, #7175, .F. ) ;
#7375=AXIS2_PLACEMENT_3D ( 'NONE', #447, #6454, #8453 ) ;
#7377=CARTESIAN_POINT ( 'NONE',  ( -49.99999999999997158, 60.00000000000002842, -30.00000000000000000 ) ) ;
#7388=ORIENTED_EDGE ( 'NONE', *, *, #3900, .F. ) ;
#7393=CARTESIAN_POINT ( 'NONE',  ( 33.30764627618177798, -48.76359959685379408, 12.05680772549332680 ) ) ;
#7398=AXIS2_PLACEMENT_3D ( 'NONE', #3657, #7711, #829 ) ;
#7405=CONICAL_SURFACE ( 'NONE', #4732, 2.099999999999997868, 1.029744258676652313 ) ;
#7419=ADVANCED_FACE ( 'NONE', ( #3902 ), #1834, .F. ) ;
#7420=VECTOR ( 'NONE', #2089, 1000.000000000000000 ) ;
#7421=DIRECTION ( 'NONE',  ( -0.000000000000000000, -0.000000000000000000, 1.000000000000000000 ) ) ;
#7442=EDGE_LOOP ( 'NONE', ( #1400, #6903, #2688 ) ) ;
#7454=CARTESIAN_POINT ( 'NONE',  ( 26.23319591279775409, -48.30383393989873042, 11.92131216183667597 ) ) ;
#7461=AXIS2_PLACEMENT_3D ( 'NONE', #6354, #5122, #4335 ) ;
#7463=CARTESIAN_POINT ( 'NONE',  ( -41.99999999999996447, 48.00000000000002842, 23.64999999999999858 ) ) ;
#7466=DIRECTION ( 'NONE',  ( -0.000000000000000000, 1.000000000000000000, -0.000000000000000000 ) ) ;
#7473=ORIENTED_EDGE ( 'NONE', *, *, #7175, .T. ) ;
#7476=CARTESIAN_POINT ( 'NONE',  ( -34.74075059544460231, -43.37701935357448946, 11.56693546130993866 ) ) ;
#7479=DIRECTION ( 'NONE',  ( 0.000000000000000000, 0.000000000000000000, 1.000000000000000000 ) ) ;
#7485=CARTESIAN_POINT ( 'NONE',  ( -49.99999999999997158, -59.99999999999997158, -30.00000000000000000 ) ) ;
#7509=ORIENTED_EDGE ( 'NONE', *, *, #2395, .T. ) ;
#7515=AXIS2_PLACEMENT_3D ( 'NONE', #1206, #1958, #2586 ) ;
#7519=CARTESIAN_POINT ( 'NONE',  ( -33.30433008846340215, -41.23356742411075260, 12.05770814628969134 ) ) ;
#7534=EDGE_CURVE ( 'NONE', #4084, #5699, #5967, .T. ) ;
#7538=FACE_OUTER_BOUND ( 'NONE', #3610, .T. ) ;
#7539=ORIENTED_EDGE ( 'NONE', *, *, #5325, .T. ) ;
#7544=AXIS2_PLACEMENT_3D ( 'NONE', #145, #2271, #2843 ) ;
#7556=AXIS2_PLACEMENT_3D ( 'NONE', #529, #620, #5212 ) ;
#7560=CARTESIAN_POINT ( 'NONE',  ( -34.96646302984643739, -44.33501760501481215, 11.47123432380333341 ) ) ;
#7562=LINE ( 'NONE', #4134, #6521 ) ;
#7563=DIRECTION ( 'NONE',  ( 0.000000000000000000, -1.000000000000000000, 0.000000000000000000 ) ) ;
#7564=EDGE_LOOP ( 'NONE', ( #6688, #5258, #4166, #5843 ) ) ;
#7568=ORIENTED_EDGE ( 'NONE', *, *, #2395, .F. ) ;
#7571=DIRECTION ( 'NONE',  ( 0.000000000000000000, 0.5150380749100549327, 0.8571673007021118895 ) ) ;
#7588=CARTESIAN_POINT ( 'NONE',  ( 27.92651295580296633, -40.44729329317335242, 12.32776405682970555 ) ) ;
#7589=DIRECTION ( 'NONE',  ( 0.000000000000000000, 0.5150380749100549327, 0.8571673007021118895 ) ) ;
#7605=EDGE_CURVE ( 'NONE', #7164, #3309, #7245, .T. ) ;
#7607=DIRECTION ( 'NONE',  ( 0.000000000000000000, 0.000000000000000000, -1.000000000000000000 ) ) ;
#7612=AXIS2_PLACEMENT_3D ( 'NONE', #349, #3057, #8432 ) ;
#7621=ADVANCED_FACE ( 'NONE', ( #8573 ), #5296, .F. ) ;
#7627=DIRECTION ( 'NONE',  ( 0.000000000000000000, 0.000000000000000000, 1.000000000000000000 ) ) ;
#7628=ADVANCED_FACE ( 'NONE', ( #6711 ), #7333, .F. ) ;
#7632=DIRECTION ( 'NONE',  ( 0.000000000000000000, 0.000000000000000000, 1.000000000000000000 ) ) ;
#7662=CONICAL_SURFACE ( 'NONE', #3865, 1.649999999999998579, 1.029744258676653645 ) ;
#7669=ADVANCED_FACE ( 'NONE', ( #3332 ), #6009, .F. ) ;
#7677=AXIS2_PLACEMENT_3D ( 'NONE', #2045, #3939, #8038 ) ;
#7696=CARTESIAN_POINT ( 'NONE',  ( 32.22816283978665552, -40.51193879865773084, 12.30361675895771967 ) ) ;
#7697=CARTESIAN_POINT ( 'NONE',  ( -30.00000000000000000, 60.00000000000002842, 0.000000000000000000 ) ) ;
#7698=CIRCLE ( 'NONE', #7255, 2.099999999999997868 ) ;
#7703=( NAMED_UNIT ( * ) PLANE_ANGLE_UNIT ( ) SI_UNIT ( $, .RADIAN. ) );
#7704=ORIENTED_EDGE ( 'NONE', *, *, #6060, .F. ) ;
#7707=CIRCLE ( 'NONE', #5872, 2.099999999999997868 ) ;
#7708=ORIENTED_EDGE ( 'NONE', *, *, #735, .T. ) ;
#7710=CARTESIAN_POINT ( 'NONE',  ( -32.23060284177036294, -49.48683715626712853, 12.30316928347423655 ) ) ;
#7711=DIRECTION ( 'NONE',  ( -0.000000000000000000, 1.000000000000000000, -0.000000000000000000 ) ) ;
#7713=LINE ( 'NONE', #1673, #2569 ) ;
#7720=ADVANCED_FACE ( 'NONE', ( #2760 ), #762, .F. ) ;
#7728=CARTESIAN_POINT ( 'NONE',  ( 45.00000000000003553, -44.99999999999997158, -2.099999999999997868 ) ) ;
#7732=ORIENTED_EDGE ( 'NONE', *, *, #3921, .T. ) ;
#7742=CARTESIAN_POINT ( 'NONE',  ( -28.37754256541759190, -49.74093594125429263, 12.39808714042240645 ) ) ;
#7752=FACE_OUTER_BOUND ( 'NONE', #4276, .T. ) ;
#7766=DIRECTION ( 'NONE',  ( 1.000000000000000000, -0.000000000000000000, -0.000000000000000000 ) ) ;
#7787=CARTESIAN_POINT ( 'NONE',  ( 0.000000000000000000, 0.000000000000000000, 0.000000000000000000 ) ) ;
#7801=ADVANCED_FACE ( 'NONE', ( #3844 ), #2661, .F. ) ;
#7802=ORIENTED_EDGE ( 'NONE', *, *, #6398, .T. ) ;
#7805=EDGE_CURVE ( 'NONE', #5614, #4623, #6568, .T. ) ;
#7828=DIRECTION ( 'NONE',  ( 0.000000000000000000, 0.000000000000000000, 1.000000000000000000 ) ) ;
#7831=SURFACE_SIDE_STYLE ('',( #4438 ) ) ;
#7837=LINE ( 'NONE', #6996, #3354 ) ;
#7840=DIRECTION ( 'NONE',  ( 0.000000000000000000, 0.5150380749100549327, 0.8571673007021118895 ) ) ;
#7845=CIRCLE ( 'NONE', #5166, 1.649999999999998579 ) ;
#7849=CYLINDRICAL_SURFACE ( 'NONE', #4653, 1.649999999999998579 ) ;
#7855=CARTESIAN_POINT ( 'NONE',  ( -41.99999999999996447, 60.00000000000002842, -22.00000000000000000 ) ) ;
#7870=CARTESIAN_POINT ( 'NONE',  ( 50.00000000000002842, -44.99999999999997158, -2.099999999999997868 ) ) ;
#7872=( NAMED_UNIT ( * ) SI_UNIT ( $, .STERADIAN. ) SOLID_ANGLE_UNIT ( ) );
#7881=CARTESIAN_POINT ( 'NONE',  ( 34.99999999999998579, -44.99999999999995737, 30.00000000000000000 ) ) ;
#7882=CARTESIAN_POINT ( 'NONE',  ( -30.00000000000002842, -57.51075773784449296, 0.000000000000000000 ) ) ;
#7884=DIRECTION ( 'NONE',  ( 0.000000000000000000, 0.000000000000000000, 1.000000000000000000 ) ) ;
#7889=ORIENTED_EDGE ( 'NONE', *, *, #7070, .F. ) ;
#7916=FACE_OUTER_BOUND ( 'NONE', #7564, .T. ) ;
#7921=AXIS2_PLACEMENT_3D ( 'NONE', #5188, #461, #5150 ) ;
#7923=CARTESIAN_POINT ( 'NONE',  ( -50.00000000000002842, -44.99999999999997158, 2.099999999999997868 ) ) ;
#7926=CARTESIAN_POINT ( 'NONE',  ( 45.00000000000003553, -44.99999999999997158, 0.000000000000000000 ) ) ;
#7936=AXIS2_PLACEMENT_3D ( 'NONE', #3690, #6413, #7081 ) ;
#7948=EDGE_CURVE ( 'NONE', #8538, #1354, #8218, .T. ) ;
#7950=CARTESIAN_POINT ( 'NONE',  ( -45.00000000000003553, -44.99999999999997158, -2.099999999999997868 ) ) ;
#7958=FACE_BOUND ( 'NONE', #897, .T. ) ;
#7969=CARTESIAN_POINT ( 'NONE',  ( 30.33389005480432132, -49.99999999999995026, 12.49999999999997158 ) ) ;
#7984=AXIS2_PLACEMENT_3D ( 'NONE', #4030, #6006, #8039 ) ;
#7998=DIRECTION ( 'NONE',  ( 1.000000000000000000, -0.000000000000000000, -0.000000000000000000 ) ) ;
#8003=ORIENTED_EDGE ( 'NONE', *, *, #6513, .F. ) ;
#8008=ADVANCED_FACE ( 'NONE', ( #7538 ), #7662, .F. ) ;
#8032=DIRECTION ( 'NONE',  ( -0.000000000000000000, -1.000000000000000000, -0.000000000000000000 ) ) ;
#8035=LINE ( 'NONE', #5, #4050 ) ;
#8038=DIRECTION ( 'NONE',  ( 0.000000000000000000, 0.000000000000000000, 1.000000000000000000 ) ) ;
#8039=DIRECTION ( 'NONE',  ( 0.000000000000000000, 0.000000000000000000, 1.000000000000000000 ) ) ;
#8041=FACE_OUTER_BOUND ( 'NONE', #550, .T. ) ;
#8046=CARTESIAN_POINT ( 'NONE',  ( 50.00000000000002842, -59.99999999999997158, 30.00000000000000000 ) ) ;
#8053=DIRECTION ( 'NONE',  ( 0.000000000000000000, 0.000000000000000000, 1.000000000000000000 ) ) ;
#8058=VERTEX_POINT ( 'NONE', #1412 ) ;
#8063=ORIENTED_EDGE ( 'NONE', *, *, #735, .F. ) ;
#8065=EDGE_CURVE ( 'NONE', #5982, #8403, #4814, .T. ) ;
#8074=VECTOR ( 'NONE', #906, 1000.000000000000000 ) ;
#8087=AXIS2_PLACEMENT_3D ( 'NONE', #4205, #7466, #1555 ) ;
#8088=DIRECTION ( 'NONE',  ( -1.000000000000000000, -0.000000000000000000, -0.000000000000000000 ) ) ;
#8089=CARTESIAN_POINT ( 'NONE',  ( 34.55267497488053863, -42.92638634940914955, 11.64163759925509822 ) ) ;
#8114=ORIENTED_EDGE ( 'NONE', *, *, #99, .F. ) ;
#8122=AXIS2_PLACEMENT_3D ( 'NONE', #4823, #846, #712 ) ;
#8125=CARTESIAN_POINT ( 'NONE',  ( 28.69346486511991046, -49.83744928702510180, 12.43572992548470246 ) ) ;
#8134=CARTESIAN_POINT ( 'NONE',  ( -25.03350713684106665, -44.33520523457838891, 11.47122145076293798 ) ) ;
#8136=DIRECTION ( 'NONE',  ( 1.000000000000000000, -0.000000000000000000, -0.000000000000000000 ) ) ;
#8146=EDGE_LOOP ( 'NONE', ( #8003, #915, #5541, #3081, #2206, #2294 ) ) ;
#8149=VERTEX_POINT ( 'NONE', #3584 ) ;
#8152=CARTESIAN_POINT ( 'NONE',  ( -32.50890011656069589, -40.67193172067895546, 12.24650812517142207 ) ) ;
#8156=ORIENTED_EDGE ( 'NONE', *, *, #803, .F. ) ;
#8159=VERTEX_POINT ( 'NONE', #883 ) ;
#8160=CARTESIAN_POINT ( 'NONE',  ( -34.99999999999997868, -45.00000000000000000, 30.00000000000000000 ) ) ;
#8165=CARTESIAN_POINT ( 'NONE',  ( -41.99999999999996447, 48.00000000000002842, 20.35000000000000142 ) ) ;
#8177=CARTESIAN_POINT ( 'NONE',  ( -29.34127574812924522, -40.04081516742419922, 12.48372095990571573 ) ) ;
#8178=CARTESIAN_POINT ( 'NONE',  ( -41.99999999999996447, 60.00000000000002842, -23.64999999999999858 ) ) ;
#8185=CARTESIAN_POINT ( 'NONE',  ( 42.00000000000000711, 60.00000000000002842, -23.64999999999992042 ) ) ;
#8194=CARTESIAN_POINT ( 'NONE',  ( 30.00000000000001421, -44.99999999999995737, 30.00000000000000000 ) ) ;
#8197=LINE ( 'NONE', #2776, #2318 ) ;
#8198=DIRECTION ( 'NONE',  ( -1.000000000000000000, 0.000000000000000000, -0.000000000000000000 ) ) ;
#8200=ORIENTED_EDGE ( 'NONE', *, *, #1018, .T. ) ;
#8204=VERTEX_POINT ( 'NONE', #1636 ) ;
#8211=AXIS2_PLACEMENT_3D ( 'NONE', #1672, #4362, #2683 ) ;
#8218=LINE ( 'NONE', #1499, #2013 ) ;
#8221=PLANE ( 'NONE',  #4821 ) ;
#8222=DIRECTION ( 'NONE',  ( 1.000000000000000000, 0.000000000000000000, 0.000000000000000000 ) ) ;
#8224=AXIS2_PLACEMENT_3D ( 'NONE', #3780, #6458, #5801 ) ;
#8225=CARTESIAN_POINT ( 'NONE',  ( -25.16324943048945073, -43.69086006543231804, 11.52652666073313092 ) ) ;
#8226=CARTESIAN_POINT ( 'NONE',  ( 30.00000000000001421, -44.99999999999995737, -30.00100000000000122 ) ) ;
#8229=CARTESIAN_POINT ( 'NONE',  ( 25.00000000000004263, -44.99999999999995737, -30.00100000000000122 ) ) ;
#8230=EDGE_LOOP ( 'NONE', ( #7388, #3638, #8200, #4005 ) ) ;
#8234=EDGE_CURVE ( 'NONE', #6235, #5482, #8302, .T. ) ;
#8241=CARTESIAN_POINT ( 'NONE',  ( 42.00000000000000711, 48.00000000000002842, -23.64999999999992042 ) ) ;
#8247=ORIENTED_EDGE ( 'NONE', *, *, #4757, .F. ) ;
#8268=CARTESIAN_POINT ( 'NONE',  ( 30.00000000000000000, 60.00000000000002842, -1.102182119232617753E-14 ) ) ;
#8276=VECTOR ( 'NONE', #728, 1000.000000000000000 ) ;
#8280=VECTOR ( 'NONE', #4226, 1000.000000000000000 ) ;
#8284=CARTESIAN_POINT ( 'NONE',  ( -25.66707447546774645, -47.51618826727541034, 11.72657454140207456 ) ) ;
#8286=ORIENTED_EDGE ( 'NONE', *, *, #7605, .F. ) ;
#8290=VERTEX_POINT ( 'NONE', #5778 ) ;
#8302=LINE ( 'NONE', #2264, #6906 ) ;
#8308=DIRECTION ( 'NONE',  ( 0.000000000000000000, 0.000000000000000000, -1.000000000000000000 ) ) ;
#8310=CARTESIAN_POINT ( 'NONE',  ( -43.73819270004214843, -44.99999999999997158, 0.000000000000000000 ) ) ;
#8314=DIRECTION ( 'NONE',  ( 1.000000000000000000, -0.000000000000000000, -0.000000000000000000 ) ) ;
#8319=AXIS2_PLACEMENT_3D ( 'NONE', #4282, #1680, #6591 ) ;
#8326=ORIENTED_EDGE ( 'NONE', *, *, #5608, .F. ) ;
#8335=DIRECTION ( 'NONE',  ( -0.000000000000000000, 1.000000000000000000, -0.000000000000000000 ) ) ;
#8340=EDGE_CURVE ( 'NONE', #8204, #8403, #6760, .T. ) ;
#8349=CIRCLE ( 'NONE', #5522, 1.649999999999998579 ) ;
#8350=ADVANCED_FACE ( 'NONE', ( #6348 ), #5734, .F. ) ;
#8359=ORIENTED_EDGE ( 'NONE', *, *, #6398, .F. ) ;
#8360=AXIS2_PLACEMENT_3D ( 'NONE', #7697, #3644, #161 ) ;
#8374=EDGE_CURVE ( 'NONE', #3309, #4035, #3260, .T. ) ;
#8375=VECTOR ( 'NONE', #7203, 1000.000000000000000 ) ;
#8380=DIRECTION ( 'NONE',  ( 1.000000000000000000, -0.000000000000000000, -0.000000000000000000 ) ) ;
#8387=ORIENTED_EDGE ( 'NONE', *, *, #1055, .T. ) ;
#8391=DIRECTION ( 'NONE',  ( 0.000000000000000000, 0.000000000000000000, -1.000000000000000000 ) ) ;
#8392=CARTESIAN_POINT ( 'NONE',  ( -45.00000000000003553, -44.99999999999997158, 2.099999999999997868 ) ) ;
#8399=CARTESIAN_POINT ( 'NONE',  ( 25.00000000000004263, -44.99999999999995737, 11.45643923738958314 ) ) ;
#8403=VERTEX_POINT ( 'NONE', #1187 ) ;
#8413=DIRECTION ( 'NONE',  ( 1.000000000000000000, 0.000000000000000000, 0.000000000000000000 ) ) ;
#8415=( NAMED_UNIT ( * ) SI_UNIT ( $, .STERADIAN. ) SOLID_ANGLE_UNIT ( ) );
#8425=DIRECTION ( 'NONE',  ( 0.000000000000000000, 0.000000000000000000, 1.000000000000000000 ) ) ;
#8432=DIRECTION ( 'NONE',  ( 0.000000000000000000, 0.000000000000000000, 1.000000000000000000 ) ) ;
#8434=CARTESIAN_POINT ( 'NONE',  ( -45.00000000000003553, -44.99999999999997158, 0.000000000000000000 ) ) ;
#8449=CARTESIAN_POINT ( 'NONE',  ( 25.00000000000004263, -44.99999999999995737, 30.00000000000000000 ) ) ;
#8450=CARTESIAN_POINT ( 'NONE',  ( 33.30788680089139575, -41.23645700522180846, 12.05676622698251776 ) ) ;
#8453=DIRECTION ( 'NONE',  ( 0.000000000000000000, 0.000000000000000000, 1.000000000000000000 ) ) ;
#8459=ORIENTED_EDGE ( 'NONE', *, *, #3755, .T. ) ;
#8468=EDGE_LOOP ( 'NONE', ( #8520, #2276 ) ) ;
#8478=FACE_OUTER_BOUND ( 'NONE', #1124, .T. ) ;
#8490=DIRECTION ( 'NONE',  ( 1.000000000000000000, -0.000000000000000000, -0.000000000000000000 ) ) ;
#8496=ADVANCED_FACE ( 'NONE', ( #8513 ), #7849, .F. ) ;
#8500=VERTEX_POINT ( 'NONE', #7312 ) ;
#8502=CARTESIAN_POINT ( 'NONE',  ( -33.05780150203954548, -48.96939036817698820, 12.12340239416035992 ) ) ;
#8505=FACE_BOUND ( 'NONE', #2022, .T. ) ;
#8513=FACE_OUTER_BOUND ( 'NONE', #8230, .T. ) ;
#8517=CYLINDRICAL_SURFACE ( 'NONE', #5199, 1.649999999999998579 ) ;
#8520=ORIENTED_EDGE ( 'NONE', *, *, #4818, .F. ) ;
#8533=SURFACE_STYLE_USAGE ( .BOTH. , #7831 ) ;
#8534=ORIENTED_EDGE ( 'NONE', *, *, #3323, .F. ) ;
#8538=VERTEX_POINT ( 'NONE', #8165 ) ;
#8539=ORIENTED_EDGE ( 'NONE', *, *, #7948, .T. ) ;
#8541=CARTESIAN_POINT ( 'NONE',  ( -31.62616360386732950, -49.73950299483296078, 12.39754634550705603 ) ) ;
#8550=VECTOR ( 'NONE', #1201, 1000.000000000000000 ) ;
#8573=FACE_OUTER_BOUND ( 'NONE', #1225, .T. ) ;
#8584=CARTESIAN_POINT ( 'NONE',  ( 34.96775378464300132, -45.65699184524252274, 11.47067790983490099 ) ) ;
#8606=EDGE_LOOP ( 'NONE', ( #3084, #6768, #5349 ) ) ;
#8613=CARTESIAN_POINT ( 'NONE',  ( 34.99999999999996447, -44.67046583110982994, 11.45643923738957426 ) ) ;
#8620=AXIS2_PLACEMENT_3D ( 'NONE', #6222, #5602, #7627 ) ;
#8630=CARTESIAN_POINT ( 'NONE',  ( 30.00000000000000000, -49.99999999999997158, -12.49999999999998046 ) ) ;
#8635=ORIENTED_EDGE ( 'NONE', *, *, #6513, .T. ) ;
#8656=CARTESIAN_POINT ( 'NONE',  ( -49.99999999999997158, -59.99999999999997158, 30.00000000000000000 ) ) ;
#8662=ORIENTED_EDGE ( 'NONE', *, *, #3777, .T. ) ;
#8668=VERTEX_POINT ( 'NONE', #7084 ) ;
#8673=CARTESIAN_POINT ( 'NONE',  ( 30.00000000000001421, -49.99999999999997158, 12.49999999999995914 ) ) ;
#8699=CARTESIAN_POINT ( 'NONE',  ( -30.00000000000000000, 60.00000000000002842, 0.000000000000000000 ) ) ;
#8701=ORIENTED_EDGE ( 'NONE', *, *, #911, .T. ) ;
ENDSEC;
END-ISO-10303-21;
